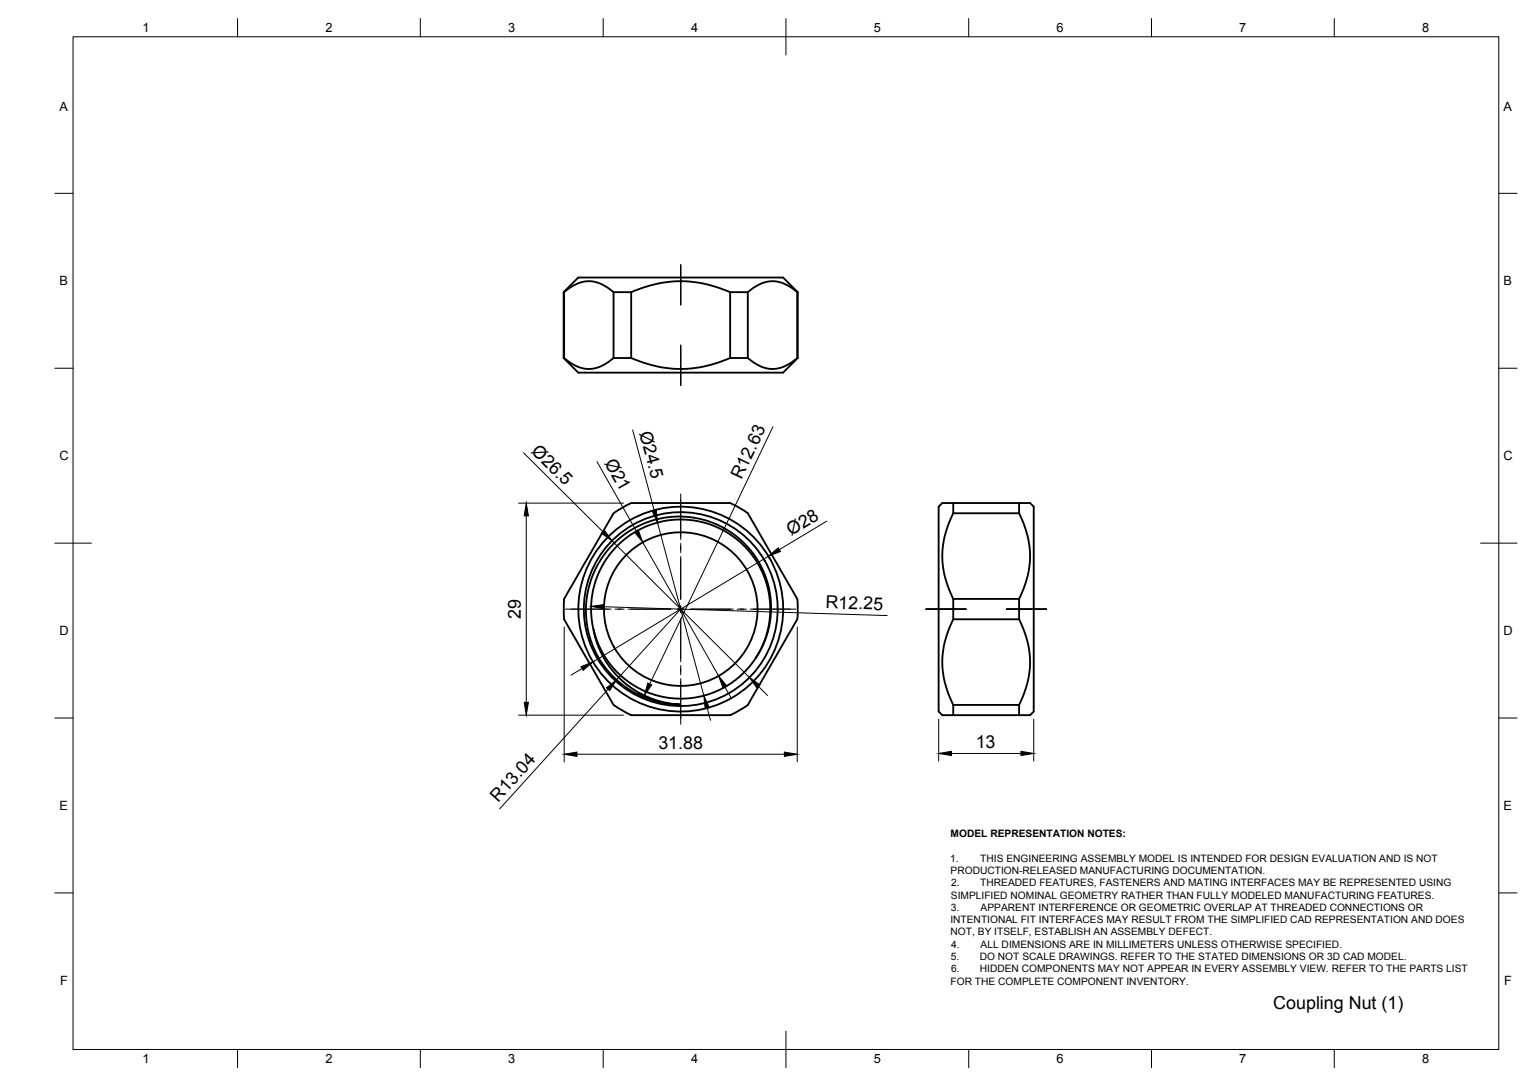
ISO-10303-21;
HEADER;
/* Generated by software containing ST-Developer
 * from STEP Tools, Inc. (www.steptools.com) 
 */

FILE_DESCRIPTION(
/* description */ ('STEP AP214'),
/* implementation_level */ '2;1');

FILE_NAME(
/* name */ 'Coupling Nut (1).step',
/* time_stamp */ '2026-10-05T23:18:41-07:00',
/* author */ (''),
/* organization */ (''),
/* preprocessor_version */ 'ST-DEVELOPER v20.2',
/* originating_system */ 'Autodesk Translation Framework v15.15.0.0',
/* authorisation */ '');

FILE_SCHEMA (('AUTOMOTIVE_DESIGN { 1 0 10303 214 3 1 1 }'));
ENDSEC;

DATA;
#10=MECHANICAL_DESIGN_GEOMETRIC_PRESENTATION_REPRESENTATION('',(#107),#221662);
#69=MANIFOLD_SOLID_BREP('Body1',#79329);
#81=SHAPE_REPRESENTATION_RELATIONSHIP('SRR','None',#221716,#94);
#94=ADVANCED_BREP_SHAPE_REPRESENTATION('',(#69),#221656);
#107=STYLED_ITEM('',(#221783),#69);
#191=B_SPLINE_SURFACE_WITH_KNOTS('',3,3,((#179610,#179611,#179612,#179613,
#179614,#179615,#179616,#179617,#179618,#179619,#179620,#179621,#179622,
#179623,#179624,#179625,#179626,#179627,#179628,#179629,#179630,#179631,
#179632,#179633,#179634,#179635,#179636,#179637,#179638,#179639,#179640,
#179641,#179642,#179643,#179644),(#179645,#179646,#179647,#179648,#179649,
#179650,#179651,#179652,#179653,#179654,#179655,#179656,#179657,#179658,
#179659,#179660,#179661,#179662,#179663,#179664,#179665,#179666,#179667,
#179668,#179669,#179670,#179671,#179672,#179673,#179674,#179675,#179676,
#179677,#179678,#179679),(#179680,#179681,#179682,#179683,#179684,#179685,
#179686,#179687,#179688,#179689,#179690,#179691,#179692,#179693,#179694,
#179695,#179696,#179697,#179698,#179699,#179700,#179701,#179702,#179703,
#179704,#179705,#179706,#179707,#179708,#179709,#179710,#179711,#179712,
#179713,#179714),(#179715,#179716,#179717,#179718,#179719,#179720,#179721,
#179722,#179723,#179724,#179725,#179726,#179727,#179728,#179729,#179730,
#179731,#179732,#179733,#179734,#179735,#179736,#179737,#179738,#179739,
#179740,#179741,#179742,#179743,#179744,#179745,#179746,#179747,#179748,
#179749)),.UNSPECIFIED.,.F.,.F.,.F.,(4,4),(4,1,1,1,1,1,1,1,1,1,1,1,1,1,
1,1,1,1,1,1,1,1,1,1,1,1,1,1,1,1,1,1,4),(0.,1.),(0.,0.031249999999992,0.062499999999984,
0.0937500000001036,0.125000000000096,0.156250000000088,0.187500000000079,
0.218750000000072,0.250000000000191,0.281250000000183,0.312500000000176,
0.343750000000167,0.375000000000159,0.406250000000151,0.437500000000271,
0.468750000000263,0.500000000000255,0.531250000000247,0.562500000000239,
0.593750000000231,0.62500000000035,0.656250000000342,0.687500000000335,
0.718750000000326,0.750000000000319,0.781250000000438,0.81250000000043,
0.843750000000422,0.875000000000414,0.906250000000406,0.937500000000398,
0.968750000000518,1.),.UNSPECIFIED.);
#192=B_SPLINE_SURFACE_WITH_KNOTS('',3,3,((#180017,#180018,#180019,#180020,
#180021,#180022,#180023,#180024,#180025,#180026,#180027,#180028,#180029,
#180030,#180031,#180032,#180033,#180034,#180035,#180036,#180037,#180038,
#180039,#180040,#180041,#180042,#180043,#180044,#180045,#180046,#180047,
#180048,#180049,#180050,#180051),(#180052,#180053,#180054,#180055,#180056,
#180057,#180058,#180059,#180060,#180061,#180062,#180063,#180064,#180065,
#180066,#180067,#180068,#180069,#180070,#180071,#180072,#180073,#180074,
#180075,#180076,#180077,#180078,#180079,#180080,#180081,#180082,#180083,
#180084,#180085,#180086),(#180087,#180088,#180089,#180090,#180091,#180092,
#180093,#180094,#180095,#180096,#180097,#180098,#180099,#180100,#180101,
#180102,#180103,#180104,#180105,#180106,#180107,#180108,#180109,#180110,
#180111,#180112,#180113,#180114,#180115,#180116,#180117,#180118,#180119,
#180120,#180121),(#180122,#180123,#180124,#180125,#180126,#180127,#180128,
#180129,#180130,#180131,#180132,#180133,#180134,#180135,#180136,#180137,
#180138,#180139,#180140,#180141,#180142,#180143,#180144,#180145,#180146,
#180147,#180148,#180149,#180150,#180151,#180152,#180153,#180154,#180155,
#180156)),.UNSPECIFIED.,.F.,.F.,.F.,(4,4),(4,1,1,1,1,1,1,1,1,1,1,1,1,1,
1,1,1,1,1,1,1,1,1,1,1,1,1,1,1,1,1,1,4),(0.,1.),(0.,0.031250000000078,0.0625000000000372,
0.0937500000001152,0.125000000000074,0.156250000000034,0.187500000000111,
0.218750000000071,0.250000000000148,0.281250000000108,0.312500000000186,
0.343750000000145,0.375000000000104,0.406250000000182,0.437500000000141,
0.468750000000219,0.500000000000178,0.531250000000256,0.562500000000216,
0.593750000000175,0.625000000000253,0.656250000000212,0.68750000000029,
0.718750000000249,0.750000000000208,0.781250000000286,0.812500000000245,
0.843750000000323,0.875000000000282,0.90625000000036,0.93750000000032,0.968750000000279,
1.),.UNSPECIFIED.);
#193=B_SPLINE_SURFACE_WITH_KNOTS('',3,3,((#180239,#180240,#180241,#180242,
#180243,#180244,#180245,#180246,#180247,#180248,#180249,#180250,#180251,
#180252,#180253,#180254,#180255,#180256,#180257,#180258,#180259,#180260,
#180261,#180262,#180263,#180264,#180265,#180266,#180267,#180268,#180269,
#180270,#180271,#180272,#180273,#180274,#180275,#180276,#180277,#180278,
#180279,#180280,#180281,#180282,#180283,#180284,#180285,#180286,#180287,
#180288,#180289,#180290,#180291,#180292,#180293,#180294,#180295,#180296,
#180297,#180298,#180299,#180300,#180301,#180302,#180303,#180304,#180305),
(#180306,#180307,#180308,#180309,#180310,#180311,#180312,#180313,#180314,
#180315,#180316,#180317,#180318,#180319,#180320,#180321,#180322,#180323,
#180324,#180325,#180326,#180327,#180328,#180329,#180330,#180331,#180332,
#180333,#180334,#180335,#180336,#180337,#180338,#180339,#180340,#180341,
#180342,#180343,#180344,#180345,#180346,#180347,#180348,#180349,#180350,
#180351,#180352,#180353,#180354,#180355,#180356,#180357,#180358,#180359,
#180360,#180361,#180362,#180363,#180364,#180365,#180366,#180367,#180368,
#180369,#180370,#180371,#180372),(#180373,#180374,#180375,#180376,#180377,
#180378,#180379,#180380,#180381,#180382,#180383,#180384,#180385,#180386,
#180387,#180388,#180389,#180390,#180391,#180392,#180393,#180394,#180395,
#180396,#180397,#180398,#180399,#180400,#180401,#180402,#180403,#180404,
#180405,#180406,#180407,#180408,#180409,#180410,#180411,#180412,#180413,
#180414,#180415,#180416,#180417,#180418,#180419,#180420,#180421,#180422,
#180423,#180424,#180425,#180426,#180427,#180428,#180429,#180430,#180431,
#180432,#180433,#180434,#180435,#180436,#180437,#180438,#180439),(#180440,
#180441,#180442,#180443,#180444,#180445,#180446,#180447,#180448,#180449,
#180450,#180451,#180452,#180453,#180454,#180455,#180456,#180457,#180458,
#180459,#180460,#180461,#180462,#180463,#180464,#180465,#180466,#180467,
#180468,#180469,#180470,#180471,#180472,#180473,#180474,#180475,#180476,
#180477,#180478,#180479,#180480,#180481,#180482,#180483,#180484,#180485,
#180486,#180487,#180488,#180489,#180490,#180491,#180492,#180493,#180494,
#180495,#180496,#180497,#180498,#180499,#180500,#180501,#180502,#180503,
#180504,#180505,#180506)),.UNSPECIFIED.,.F.,.F.,.F.,(4,4),(4,1,1,1,1,1,
1,1,1,1,1,1,1,1,1,1,1,1,1,1,1,1,1,1,1,1,1,1,1,1,1,1,1,1,1,1,1,1,1,1,1,1,
1,1,1,1,1,1,1,1,1,1,1,1,1,1,1,1,1,1,1,1,1,1,4),(0.,1.),(0.,0.015625,0.03125,
0.046875,0.0625,0.078125,0.09375,0.109375,0.125,0.140625,0.15625,0.171875,
0.1875,0.203125,0.21875,0.234375,0.25,0.265625,0.28125,0.296875,0.3125,
0.328125,0.34375,0.359375,0.375,0.390625,0.40625,0.421875,0.4375,0.453125,
0.46875,0.484375,0.5,0.515625,0.53125,0.546875,0.5625,0.578125,0.59375,
0.609375,0.625,0.640625,0.65625,0.671875,0.6875,0.703125,0.71875,0.734375,
0.75,0.765625,0.78125,0.796875,0.8125,0.828125,0.84375,0.859375,0.875,0.890625,
0.90625,0.921875,0.9375,0.953125,0.96875,0.984375,1.),.UNSPECIFIED.);
#194=B_SPLINE_SURFACE_WITH_KNOTS('',3,3,((#180514,#180515,#180516,#180517,
#180518),(#180519,#180520,#180521,#180522,#180523),(#180524,#180525,#180526,
#180527,#180528),(#180529,#180530,#180531,#180532,#180533)),
 .UNSPECIFIED.,.F.,.F.,.F.,(4,4),(4,1,4),(0.,1.),(0.,0.500000000000012,
1.),.UNSPECIFIED.);
#195=B_SPLINE_SURFACE_WITH_KNOTS('',3,1,((#180592,#180593),(#180594,#180595),
(#180596,#180597),(#180598,#180599),(#180600,#180601),(#180602,#180603),
(#180604,#180605),(#180606,#180607),(#180608,#180609),(#180610,#180611),
(#180612,#180613),(#180614,#180615)),.UNSPECIFIED.,.F.,.F.,.F.,(4,2,2,2,
2,4),(2,2),(0.0140497253938089,0.25,0.5,0.75,0.875,0.987103459251385),(0.,
0.0717898562567659),.UNSPECIFIED.);
#196=B_SPLINE_SURFACE_WITH_KNOTS('',3,3,((#180674,#180675,#180676,#180677,
#180678),(#180679,#180680,#180681,#180682,#180683),(#180684,#180685,#180686,
#180687,#180688),(#180689,#180690,#180691,#180692,#180693)),
 .UNSPECIFIED.,.F.,.F.,.F.,(4,4),(4,1,4),(0.,1.),(0.,0.500000000000012,
1.),.UNSPECIFIED.);
#197=B_SPLINE_SURFACE_WITH_KNOTS('',3,3,((#180700,#180701,#180702,#180703,
#180704,#180705,#180706,#180707,#180708,#180709,#180710,#180711,#180712,
#180713,#180714,#180715,#180716,#180717,#180718,#180719,#180720,#180721,
#180722,#180723,#180724,#180725,#180726,#180727,#180728,#180729,#180730,
#180731,#180732,#180733,#180734,#180735,#180736,#180737,#180738,#180739,
#180740,#180741,#180742,#180743,#180744,#180745,#180746,#180747,#180748,
#180749,#180750,#180751,#180752,#180753,#180754,#180755,#180756,#180757,
#180758,#180759,#180760,#180761,#180762,#180763,#180764,#180765,#180766),
(#180767,#180768,#180769,#180770,#180771,#180772,#180773,#180774,#180775,
#180776,#180777,#180778,#180779,#180780,#180781,#180782,#180783,#180784,
#180785,#180786,#180787,#180788,#180789,#180790,#180791,#180792,#180793,
#180794,#180795,#180796,#180797,#180798,#180799,#180800,#180801,#180802,
#180803,#180804,#180805,#180806,#180807,#180808,#180809,#180810,#180811,
#180812,#180813,#180814,#180815,#180816,#180817,#180818,#180819,#180820,
#180821,#180822,#180823,#180824,#180825,#180826,#180827,#180828,#180829,
#180830,#180831,#180832,#180833),(#180834,#180835,#180836,#180837,#180838,
#180839,#180840,#180841,#180842,#180843,#180844,#180845,#180846,#180847,
#180848,#180849,#180850,#180851,#180852,#180853,#180854,#180855,#180856,
#180857,#180858,#180859,#180860,#180861,#180862,#180863,#180864,#180865,
#180866,#180867,#180868,#180869,#180870,#180871,#180872,#180873,#180874,
#180875,#180876,#180877,#180878,#180879,#180880,#180881,#180882,#180883,
#180884,#180885,#180886,#180887,#180888,#180889,#180890,#180891,#180892,
#180893,#180894,#180895,#180896,#180897,#180898,#180899,#180900),(#180901,
#180902,#180903,#180904,#180905,#180906,#180907,#180908,#180909,#180910,
#180911,#180912,#180913,#180914,#180915,#180916,#180917,#180918,#180919,
#180920,#180921,#180922,#180923,#180924,#180925,#180926,#180927,#180928,
#180929,#180930,#180931,#180932,#180933,#180934,#180935,#180936,#180937,
#180938,#180939,#180940,#180941,#180942,#180943,#180944,#180945,#180946,
#180947,#180948,#180949,#180950,#180951,#180952,#180953,#180954,#180955,
#180956,#180957,#180958,#180959,#180960,#180961,#180962,#180963,#180964,
#180965,#180966,#180967)),.UNSPECIFIED.,.F.,.F.,.F.,(4,4),(4,1,1,1,1,1,
1,1,1,1,1,1,1,1,1,1,1,1,1,1,1,1,1,1,1,1,1,1,1,1,1,1,1,1,1,1,1,1,1,1,1,1,
1,1,1,1,1,1,1,1,1,1,1,1,1,1,1,1,1,1,1,1,1,1,4),(0.,1.),(0.,0.015625,0.03125,
0.046875,0.0625,0.078125,0.09375,0.109375,0.125,0.140625,0.15625,0.171875,
0.1875,0.203125,0.21875,0.234375,0.25,0.265625,0.28125,0.296875,0.3125,
0.328125,0.34375,0.359375,0.375,0.390625,0.40625,0.421875,0.4375,0.453125,
0.46875,0.484375,0.5,0.515625,0.53125,0.546875,0.5625,0.578125,0.59375,
0.609375,0.625,0.640625,0.65625,0.671875,0.6875,0.703125,0.71875,0.734375,
0.75,0.765625,0.78125,0.796875,0.8125,0.828125,0.84375,0.859375,0.875,0.890625,
0.90625,0.921875,0.9375,0.953125,0.96875,0.984375,1.),.UNSPECIFIED.);
#198=B_SPLINE_SURFACE_WITH_KNOTS('',3,3,((#180968,#180969,#180970,#180971,
#180972,#180973,#180974,#180975,#180976,#180977,#180978,#180979,#180980,
#180981,#180982,#180983,#180984,#180985,#180986,#180987,#180988,#180989,
#180990,#180991,#180992,#180993,#180994,#180995,#180996,#180997,#180998,
#180999,#181000,#181001,#181002),(#181003,#181004,#181005,#181006,#181007,
#181008,#181009,#181010,#181011,#181012,#181013,#181014,#181015,#181016,
#181017,#181018,#181019,#181020,#181021,#181022,#181023,#181024,#181025,
#181026,#181027,#181028,#181029,#181030,#181031,#181032,#181033,#181034,
#181035,#181036,#181037),(#181038,#181039,#181040,#181041,#181042,#181043,
#181044,#181045,#181046,#181047,#181048,#181049,#181050,#181051,#181052,
#181053,#181054,#181055,#181056,#181057,#181058,#181059,#181060,#181061,
#181062,#181063,#181064,#181065,#181066,#181067,#181068,#181069,#181070,
#181071,#181072),(#181073,#181074,#181075,#181076,#181077,#181078,#181079,
#181080,#181081,#181082,#181083,#181084,#181085,#181086,#181087,#181088,
#181089,#181090,#181091,#181092,#181093,#181094,#181095,#181096,#181097,
#181098,#181099,#181100,#181101,#181102,#181103,#181104,#181105,#181106,
#181107)),.UNSPECIFIED.,.F.,.F.,.F.,(4,4),(4,1,1,1,1,1,1,1,1,1,1,1,1,1,
1,1,1,1,1,1,1,1,1,1,1,1,1,1,1,1,1,1,4),(0.,1.),(0.,0.031250000000078,0.0625000000000372,
0.0937500000001152,0.125000000000074,0.156250000000034,0.187500000000111,
0.218750000000071,0.250000000000148,0.281250000000108,0.312500000000186,
0.343750000000145,0.375000000000104,0.406250000000182,0.437500000000141,
0.468750000000219,0.500000000000178,0.531250000000256,0.562500000000216,
0.593750000000175,0.625000000000253,0.656250000000212,0.68750000000029,
0.718750000000249,0.750000000000208,0.781250000000286,0.812500000000245,
0.843750000000323,0.875000000000282,0.90625000000036,0.93750000000032,0.968750000000279,
1.),.UNSPECIFIED.);
#302=FACE_BOUND('',#24853,.T.);
#303=FACE_BOUND('',#24863,.T.);
#304=FACE_BOUND('',#24865,.T.);
#1788=(
BOUNDED_CURVE()
B_SPLINE_CURVE(2,(#179504,#179505,#179506),.UNSPECIFIED.,.F.,.F.)
B_SPLINE_CURVE_WITH_KNOTS((3,3),(1.60808462077176,3.73981215786377),
 .UNSPECIFIED.)
CURVE()
GEOMETRIC_REPRESENTATION_ITEM()
RATIONAL_B_SPLINE_CURVE((1.37704917963476,1.51950254302061,1.37704917962903))
REPRESENTATION_ITEM('')
);
#1789=(
BOUNDED_CURVE()
B_SPLINE_CURVE(2,(#179510,#179511,#179512),.UNSPECIFIED.,.F.,.F.)
B_SPLINE_CURVE_WITH_KNOTS((3,3),(1.608096434994,3.73983031850901),
 .UNSPECIFIED.)
CURVE()
GEOMETRIC_REPRESENTATION_ITEM()
RATIONAL_B_SPLINE_CURVE((1.37705242397046,1.51950612297584,1.37705242396616))
REPRESENTATION_ITEM('')
);
#1790=(
BOUNDED_CURVE()
B_SPLINE_CURVE(2,(#179516,#179517,#179518),.UNSPECIFIED.,.F.,.F.)
B_SPLINE_CURVE_WITH_KNOTS((3,3),(-3.73983031850899,-1.60809643499399),
 .UNSPECIFIED.)
CURVE()
GEOMETRIC_REPRESENTATION_ITEM()
RATIONAL_B_SPLINE_CURVE((1.37705242396616,1.51950612297584,1.37705242397046))
REPRESENTATION_ITEM('')
);
#1791=(
BOUNDED_CURVE()
B_SPLINE_CURVE(2,(#179522,#179523,#179524),.UNSPECIFIED.,.F.,.F.)
B_SPLINE_CURVE_WITH_KNOTS((3,3),(1.60808462077176,3.73981215785304),
 .UNSPECIFIED.)
CURVE()
GEOMETRIC_REPRESENTATION_ITEM()
RATIONAL_B_SPLINE_CURVE((1.37704917963476,1.51950254301988,1.37704917963046))
REPRESENTATION_ITEM('')
);
#1792=(
BOUNDED_CURVE()
B_SPLINE_CURVE(2,(#179528,#179529,#179530),.UNSPECIFIED.,.F.,.F.)
B_SPLINE_CURVE_WITH_KNOTS((3,3),(1.60809643499362,3.73983031850844),
 .UNSPECIFIED.)
CURVE()
GEOMETRIC_REPRESENTATION_ITEM()
RATIONAL_B_SPLINE_CURVE((1.37705242397036,1.51950612297573,1.37705242396606))
REPRESENTATION_ITEM('')
);
#1793=(
BOUNDED_CURVE()
B_SPLINE_CURVE(2,(#179539,#179540,#179541),.UNSPECIFIED.,.F.,.F.)
B_SPLINE_CURVE_WITH_KNOTS((3,3),(1.60809643499432,3.73983031850951),
 .UNSPECIFIED.)
CURVE()
GEOMETRIC_REPRESENTATION_ITEM()
RATIONAL_B_SPLINE_CURVE((1.37705242397056,1.51950612297595,1.37705242396626))
REPRESENTATION_ITEM('')
);
#1794=(
BOUNDED_CURVE()
B_SPLINE_CURVE(2,(#179546,#179547,#179548),.UNSPECIFIED.,.F.,.F.)
B_SPLINE_CURVE_WITH_KNOTS((3,3),(1.76947846838519,3.98831685496984),
 .UNSPECIFIED.)
CURVE()
GEOMETRIC_REPRESENTATION_ITEM()
RATIONAL_B_SPLINE_CURVE((1.4216188517591,1.56868287088004,1.4216188517602))
REPRESENTATION_ITEM('')
);
#1795=(
BOUNDED_CURVE()
B_SPLINE_CURVE(2,(#179552,#179553,#179554),.UNSPECIFIED.,.F.,.F.)
B_SPLINE_CURVE_WITH_KNOTS((3,3),(-3.98831685495251,-1.76947846838546),
 .UNSPECIFIED.)
CURVE()
GEOMETRIC_REPRESENTATION_ITEM()
RATIONAL_B_SPLINE_CURVE((1.42161885176135,1.56868287087821,1.42161885175877))
REPRESENTATION_ITEM('')
);
#1796=(
BOUNDED_CURVE()
B_SPLINE_CURVE(2,(#179558,#179559,#179560),.UNSPECIFIED.,.F.,.F.)
B_SPLINE_CURVE_WITH_KNOTS((3,3),(1.76947846838545,3.98831685495252),
 .UNSPECIFIED.)
CURVE()
GEOMETRIC_REPRESENTATION_ITEM()
RATIONAL_B_SPLINE_CURVE((1.42161885175877,1.56868287087821,1.42161885176135))
REPRESENTATION_ITEM('')
);
#1797=(
BOUNDED_CURVE()
B_SPLINE_CURVE(2,(#179564,#179565,#179566),.UNSPECIFIED.,.F.,.F.)
B_SPLINE_CURVE_WITH_KNOTS((3,3),(1.76947846838366,3.98831685496743),
 .UNSPECIFIED.)
CURVE()
GEOMETRIC_REPRESENTATION_ITEM()
RATIONAL_B_SPLINE_CURVE((1.42161885175867,1.56868287087956,1.42161885175977))
REPRESENTATION_ITEM('')
);
#1798=(
BOUNDED_CURVE()
B_SPLINE_CURVE(2,(#179570,#179571,#179572),.UNSPECIFIED.,.F.,.F.)
B_SPLINE_CURVE_WITH_KNOTS((3,3),(-3.98831685495253,-1.76947846838542),
 .UNSPECIFIED.)
CURVE()
GEOMETRIC_REPRESENTATION_ITEM()
RATIONAL_B_SPLINE_CURVE((1.42161885176134,1.56868287087821,1.42161885175876))
REPRESENTATION_ITEM('')
);
#1799=(
BOUNDED_CURVE()
B_SPLINE_CURVE(2,(#179581,#179582,#179583),.UNSPECIFIED.,.F.,.F.)
B_SPLINE_CURVE_WITH_KNOTS((3,3),(-3.98831685495253,-1.76947846838542),
 .UNSPECIFIED.)
CURVE()
GEOMETRIC_REPRESENTATION_ITEM()
RATIONAL_B_SPLINE_CURVE((1.42161885176135,1.56868287087821,1.42161885175877))
REPRESENTATION_ITEM('')
);
#1944=CONICAL_SURFACE('',#80813,12.750003108,0.785398266415682);
#1945=CONICAL_SURFACE('',#80815,15.,0.7853981625);
#1946=CONICAL_SURFACE('',#80824,15.,0.7853981625);
#2237=CYLINDRICAL_SURFACE('',#80797,13.0486498132185);
#2238=CYLINDRICAL_SURFACE('',#80798,13.0486498132185);
#2239=CYLINDRICAL_SURFACE('',#80799,13.0486498132185);
#2240=CYLINDRICAL_SURFACE('',#80800,12.25);
#2241=CYLINDRICAL_SURFACE('',#80802,12.25);
#2242=CYLINDRICAL_SURFACE('',#80803,12.25);
#2243=CYLINDRICAL_SURFACE('',#80804,12.25);
#2244=CYLINDRICAL_SURFACE('',#80805,12.25);
#2245=CYLINDRICAL_SURFACE('',#80807,10.5);
#2246=CYLINDRICAL_SURFACE('',#80810,12.25);
#2247=CYLINDRICAL_SURFACE('',#80812,13.0486498132185);
#2248=CYLINDRICAL_SURFACE('',#80833,16.);
#2249=CYLINDRICAL_SURFACE('',#80837,16.);
#2250=CYLINDRICAL_SURFACE('',#80838,16.);
#2251=CYLINDRICAL_SURFACE('',#80841,16.);
#2252=CYLINDRICAL_SURFACE('',#80842,16.);
#2253=CYLINDRICAL_SURFACE('',#80843,16.);
#3159=LINE('',#177999,#10226);
#3160=LINE('',#178079,#10227);
#3161=LINE('',#178155,#10228);
#3162=LINE('',#178321,#10229);
#3163=LINE('',#178351,#10230);
#3164=LINE('',#178420,#10231);
#3165=LINE('',#178487,#10232);
#3166=LINE('',#178570,#10233);
#3167=LINE('',#178736,#10234);
#3168=LINE('',#178905,#10235);
#3169=LINE('',#179064,#10236);
#3170=LINE('',#179079,#10237);
#3171=LINE('',#179394,#10238);
#3172=LINE('',#179534,#10239);
#3173=LINE('',#179576,#10240);
#3174=LINE('',#179586,#10241);
#3175=LINE('',#179587,#10242);
#3176=LINE('',#179589,#10243);
#3177=LINE('',#179590,#10244);
#3178=LINE('',#179592,#10245);
#3179=LINE('',#179594,#10246);
#3180=LINE('',#179596,#10247);
#3181=LINE('',#179598,#10248);
#3182=LINE('',#179600,#10249);
#3183=LINE('',#179602,#10250);
#3184=LINE('',#179603,#10251);
#3185=LINE('',#179606,#10252);
#3186=LINE('',#180016,#10253);
#3187=LINE('',#180513,#10254);
#10226=VECTOR('',#89254,13.0486498132185);
#10227=VECTOR('',#89255,10.);
#10228=VECTOR('',#89258,13.0486498132185);
#10229=VECTOR('',#89261,13.0486498132185);
#10230=VECTOR('',#89264,12.25);
#10231=VECTOR('',#89265,10.);
#10232=VECTOR('',#89266,12.25);
#10233=VECTOR('',#89271,12.25);
#10234=VECTOR('',#89274,12.25);
#10235=VECTOR('',#89277,12.25);
#10236=VECTOR('',#89280,12.25);
#10237=VECTOR('',#89287,10.5);
#10238=VECTOR('',#89298,12.750003108);
#10239=VECTOR('',#89313,15.);
#10240=VECTOR('',#89332,15.);
#10241=VECTOR('',#89341,1000.);
#10242=VECTOR('',#89342,1000.);
#10243=VECTOR('',#89345,1000.);
#10244=VECTOR('',#89346,1000.);
#10245=VECTOR('',#89349,1000.);
#10246=VECTOR('',#89352,1000.);
#10247=VECTOR('',#89355,1000.);
#10248=VECTOR('',#89358,1000.);
#10249=VECTOR('',#89361,1000.);
#10250=VECTOR('',#89364,1000.);
#10251=VECTOR('',#89365,1000.);
#10252=VECTOR('',#89370,1000.);
#10253=VECTOR('',#89377,10.);
#10254=VECTOR('',#89378,10.);
#16994=PLANE('',#80834);
#16995=PLANE('',#80835);
#16996=PLANE('',#80836);
#16997=PLANE('',#80839);
#16998=PLANE('',#80840);
#16999=PLANE('',#80844);
#17000=PLANE('',#80845);
#17001=PLANE('',#80846);
#17002=PLANE('',#80847);
#20754=FACE_OUTER_BOUND('',#24826,.T.);
#20755=FACE_OUTER_BOUND('',#24827,.T.);
#20756=FACE_OUTER_BOUND('',#24828,.T.);
#20757=FACE_OUTER_BOUND('',#24829,.T.);
#20758=FACE_OUTER_BOUND('',#24830,.T.);
#20759=FACE_OUTER_BOUND('',#24831,.T.);
#20760=FACE_OUTER_BOUND('',#24832,.T.);
#20761=FACE_OUTER_BOUND('',#24833,.T.);
#20762=FACE_OUTER_BOUND('',#24834,.T.);
#20763=FACE_OUTER_BOUND('',#24835,.T.);
#20764=FACE_OUTER_BOUND('',#24836,.T.);
#20765=FACE_OUTER_BOUND('',#24837,.T.);
#20766=FACE_OUTER_BOUND('',#24838,.T.);
#20767=FACE_OUTER_BOUND('',#24839,.T.);
#20768=FACE_OUTER_BOUND('',#24840,.T.);
#20769=FACE_OUTER_BOUND('',#24841,.T.);
#20770=FACE_OUTER_BOUND('',#24842,.T.);
#20771=FACE_OUTER_BOUND('',#24843,.T.);
#20772=FACE_OUTER_BOUND('',#24844,.T.);
#20773=FACE_OUTER_BOUND('',#24845,.T.);
#20774=FACE_OUTER_BOUND('',#24846,.T.);
#20775=FACE_OUTER_BOUND('',#24847,.T.);
#20776=FACE_OUTER_BOUND('',#24848,.T.);
#20777=FACE_OUTER_BOUND('',#24849,.T.);
#20778=FACE_OUTER_BOUND('',#24850,.T.);
#20779=FACE_OUTER_BOUND('',#24851,.T.);
#20780=FACE_OUTER_BOUND('',#24852,.T.);
#20781=FACE_OUTER_BOUND('',#24854,.T.);
#20782=FACE_OUTER_BOUND('',#24855,.T.);
#20783=FACE_OUTER_BOUND('',#24856,.T.);
#20784=FACE_OUTER_BOUND('',#24857,.T.);
#20785=FACE_OUTER_BOUND('',#24858,.T.);
#20786=FACE_OUTER_BOUND('',#24859,.T.);
#20787=FACE_OUTER_BOUND('',#24860,.T.);
#20788=FACE_OUTER_BOUND('',#24861,.T.);
#20789=FACE_OUTER_BOUND('',#24862,.T.);
#20790=FACE_OUTER_BOUND('',#24864,.T.);
#24826=EDGE_LOOP('',(#56697,#56698,#56699,#56700,#56701));
#24827=EDGE_LOOP('',(#56702,#56703,#56704,#56705));
#24828=EDGE_LOOP('',(#56706,#56707,#56708,#56709));
#24829=EDGE_LOOP('',(#56710,#56711,#56712,#56713,#56714,#56715,#56716,#56717,
#56718,#56719,#56720,#56721));
#24830=EDGE_LOOP('',(#56722,#56723,#56724,#56725));
#24831=EDGE_LOOP('',(#56726,#56727,#56728,#56729,#56730));
#24832=EDGE_LOOP('',(#56731,#56732,#56733,#56734,#56735));
#24833=EDGE_LOOP('',(#56736,#56737,#56738));
#24834=EDGE_LOOP('',(#56739,#56740,#56741,#56742));
#24835=EDGE_LOOP('',(#56743,#56744,#56745,#56746,#56747,#56748));
#24836=EDGE_LOOP('',(#56749,#56750,#56751,#56752));
#24837=EDGE_LOOP('',(#56753,#56754,#56755,#56756,#56757,#56758,#56759,#56760,
#56761,#56762));
#24838=EDGE_LOOP('',(#56763,#56764,#56765,#56766,#56767,#56768,#56769,#56770,
#56771,#56772,#56773,#56774,#56775,#56776,#56777,#56778));
#24839=EDGE_LOOP('',(#56779,#56780,#56781,#56782,#56783,#56784,#56785,#56786,
#56787,#56788,#56789,#56790,#56791,#56792,#56793,#56794));
#24840=EDGE_LOOP('',(#56795,#56796,#56797,#56798,#56799));
#24841=EDGE_LOOP('',(#56800,#56801,#56802,#56803));
#24842=EDGE_LOOP('',(#56804,#56805,#56806,#56807));
#24843=EDGE_LOOP('',(#56808,#56809,#56810,#56811));
#24844=EDGE_LOOP('',(#56812,#56813,#56814,#56815));
#24845=EDGE_LOOP('',(#56816,#56817,#56818,#56819));
#24846=EDGE_LOOP('',(#56820,#56821,#56822,#56823));
#24847=EDGE_LOOP('',(#56824,#56825,#56826,#56827));
#24848=EDGE_LOOP('',(#56828,#56829,#56830,#56831));
#24849=EDGE_LOOP('',(#56832,#56833,#56834,#56835));
#24850=EDGE_LOOP('',(#56836,#56837,#56838,#56839,#56840));
#24851=EDGE_LOOP('',(#56841,#56842,#56843,#56844));
#24852=EDGE_LOOP('',(#56845));
#24853=EDGE_LOOP('',(#56846));
#24854=EDGE_LOOP('',(#56847,#56848,#56849,#56850,#56851,#56852,#56853));
#24855=EDGE_LOOP('',(#56854,#56855,#56856,#56857,#56858));
#24856=EDGE_LOOP('',(#56859,#56860,#56861,#56862,#56863,#56864,#56865,#56866,
#56867,#56868,#56869));
#24857=EDGE_LOOP('',(#56870,#56871,#56872));
#24858=EDGE_LOOP('',(#56873,#56874,#56875,#56876));
#24859=EDGE_LOOP('',(#56877,#56878,#56879));
#24860=EDGE_LOOP('',(#56880,#56881,#56882,#56883,#56884,#56885,#56886,#56887,
#56888,#56889,#56890,#56891));
#24861=EDGE_LOOP('',(#56892,#56893,#56894,#56895,#56896,#56897,#56898));
#24862=EDGE_LOOP('',(#56899));
#24863=EDGE_LOOP('',(#56900));
#24864=EDGE_LOOP('',(#56901));
#24865=EDGE_LOOP('',(#56902));
#30234=B_SPLINE_CURVE_WITH_KNOTS('',3,(#178001,#178002,#178003,#178004,
#178005,#178006,#178007,#178008,#178009,#178010,#178011,#178012,#178013,
#178014,#178015,#178016,#178017,#178018,#178019,#178020,#178021,#178022,
#178023,#178024,#178025,#178026,#178027,#178028,#178029,#178030,#178031,
#178032,#178033,#178034,#178035,#178036,#178037,#178038,#178039,#178040,
#178041,#178042),.UNSPECIFIED.,.F.,.F.,(4,2,2,2,2,2,2,2,2,2,2,2,2,2,2,2,
2,2,2,2,4),(16.411939559148,16.5276993648978,16.7898103993412,16.9146234716417,
17.1336164713817,17.331869283095,17.5558277390514,17.7571272017244,17.9098817122033,
18.1686635086661,18.3330413380558,18.5331993144161,18.7925278924566,19.0512622565918,
19.1783118587244,19.3819635677508,19.6487024603407,19.7552464035092,20.0145823158284,
20.2601584579687,20.5148551545717),.UNSPECIFIED.);
#30235=B_SPLINE_CURVE_WITH_KNOTS('',3,(#178044,#178045,#178046,#178047,
#178048,#178049,#178050,#178051,#178052,#178053,#178054,#178055,#178056,
#178057,#178058,#178059,#178060,#178061,#178062,#178063,#178064,#178065,
#178066,#178067,#178068,#178069,#178070,#178071,#178072,#178073,#178074,
#178075,#178076,#178077),.UNSPECIFIED.,.F.,.F.,(4,2,2,2,2,2,2,2,2,2,2,2,
2,2,2,2,4),(-3.64743130453341,-3.33257853567476,-3.22780382457832,-2.94609671661996,
-2.68640335637872,-2.43382900975111,-2.07865629233289,-1.823297444294,-1.69779781578983,
-1.49131358643798,-1.2705775614283,-1.11563261310354,-0.884376073702807,
-0.690814598996595,-0.518873862852227,-0.260515535699254,-0.000141823912015393),
 .UNSPECIFIED.);
#30236=B_SPLINE_CURVE_WITH_KNOTS('',3,(#178080,#178081,#178082,#178083,
#178084,#178085,#178086,#178087,#178088,#178089,#178090,#178091,#178092,
#178093,#178094,#178095,#178096,#178097,#178098,#178099,#178100,#178101,
#178102,#178103,#178104,#178105,#178106,#178107,#178108,#178109,#178110,
#178111,#178112,#178113,#178114,#178115,#178116,#178117,#178118,#178119,
#178120,#178121,#178122,#178123,#178124,#178125,#178126,#178127,#178128,
#178129,#178130,#178131,#178132,#178133,#178134,#178135,#178136,#178137,
#178138,#178139,#178140,#178141,#178142,#178143,#178144,#178145,#178146,
#178147,#178148,#178149,#178150,#178151),.UNSPECIFIED.,.F.,.F.,(4,2,2,2,
2,2,2,2,2,2,2,2,2,2,2,2,2,2,2,2,2,2,2,2,2,2,2,2,2,2,2,2,2,2,2,4),(0.000165493788789278,
0.133572515359782,0.265070417066448,0.525261541659564,0.718250836461765,
0.939262619734119,1.10101308860442,1.36078600247732,1.61438552821345,1.86608480335074,
2.10918592858206,2.36534540858103,2.49037418921662,2.71408475481147,2.97308494587933,
3.09890243561411,3.35779973017724,3.57542031480175,3.79208623060398,4.04882373567806,
4.30051979229931,4.55920852636254,4.81123563101406,5.01845678813855,5.27455044290403,
5.52645653972308,5.76250743234395,6.00874266289446,6.20633919438028,6.3337050145735,
6.59244105306261,6.85126540653577,7.05793450067292,7.31164686257427,7.56543499053437,
7.75024417698323),.UNSPECIFIED.);
#30237=B_SPLINE_CURVE_WITH_KNOTS('',3,(#178156,#178157,#178158,#178159,
#178160,#178161,#178162,#178163,#178164,#178165,#178166,#178167,#178168,
#178169,#178170,#178171,#178172,#178173,#178174,#178175,#178176,#178177,
#178178,#178179,#178180,#178181,#178182,#178183,#178184,#178185,#178186,
#178187,#178188,#178189,#178190,#178191,#178192,#178193,#178194,#178195,
#178196,#178197,#178198,#178199,#178200,#178201,#178202,#178203,#178204,
#178205,#178206,#178207,#178208,#178209,#178210,#178211,#178212,#178213,
#178214,#178215,#178216,#178217,#178218,#178219,#178220,#178221,#178222,
#178223,#178224,#178225,#178226,#178227,#178228,#178229,#178230,#178231,
#178232,#178233,#178234,#178235,#178236,#178237),.UNSPECIFIED.,.F.,.F.,
(4,2,2,2,2,2,2,2,2,2,2,2,2,2,2,2,2,2,2,2,2,2,2,2,2,2,2,2,2,2,2,2,2,2,2,
2,2,2,2,2,4),(8.20599054997932,8.35079045388701,8.60924481411329,8.75465398952731,
8.95626211349646,9.21554237835956,9.34443315214084,9.58153550224463,9.77860946937124,
10.0041117166618,10.2579350567844,10.3824872891584,10.6879416879749,10.8130137052272,
11.0351748170972,11.2420075009466,11.4004731687472,11.6129596147629,11.8470240825678,
12.0601025163729,12.2237306704323,12.4823623009414,12.6947479399234,12.8195512556543,
13.0784335443201,13.3076522799465,13.4323904647595,13.6664221203585,13.8636547400886,
14.0842574617044,14.3120516628972,14.5550127212924,14.8073205727347,15.0605117862674,
15.3202978529829,15.4883699770317,15.7022609398385,15.8985108557244,16.1077929373567,
16.3226600726361,16.411939559148),.UNSPECIFIED.);
#30238=B_SPLINE_CURVE_WITH_KNOTS('',3,(#178238,#178239,#178240,#178241,
#178242,#178243,#178244,#178245,#178246,#178247,#178248,#178249,#178250,
#178251,#178252,#178253,#178254,#178255,#178256,#178257,#178258,#178259,
#178260,#178261,#178262,#178263,#178264,#178265,#178266,#178267,#178268,
#178269,#178270,#178271,#178272,#178273,#178274,#178275,#178276,#178277,
#178278,#178279,#178280,#178281,#178282,#178283,#178284,#178285,#178286,
#178287,#178288,#178289,#178290,#178291,#178292,#178293,#178294,#178295,
#178296,#178297,#178298,#178299,#178300,#178301,#178302,#178303,#178304,
#178305,#178306,#178307,#178308,#178309,#178310,#178311,#178312,#178313,
#178314,#178315,#178316,#178317),.UNSPECIFIED.,.F.,.F.,(4,2,2,2,2,2,2,2,
2,2,2,2,2,2,2,2,2,2,2,2,2,2,2,2,2,2,2,2,2,2,2,2,2,2,2,2,2,2,2,4),(7.75024417698323,
7.82451593103171,8.02113898697175,8.28067309482283,8.53374289089235,8.78755898378574,
9.04712635066033,9.26728651955331,9.48617872391405,9.68037806711142,9.90991948493791,
10.0351210994055,10.2947590347315,10.4947121782736,10.7212623316305,10.8466717851503,
11.1058046174447,11.3157786202329,11.5462098319442,11.6980972601113,11.9564972275347,
12.0809855194537,12.3324431280832,12.5428274659398,12.7594848200696,13.0187426511126,
13.2711191413954,13.5240636571919,13.7831182451389,13.9451540287318,14.1483747254047,
14.4416992472351,14.5664190762602,14.7966381602951,14.9957380443166,15.260658195038,
15.3855066671222,15.5901676955325,15.848864838421,15.9563811041735),
 .UNSPECIFIED.);
#30239=B_SPLINE_CURVE_WITH_KNOTS('',3,(#178323,#178324,#178325,#178326,
#178327,#178328,#178329,#178330,#178331,#178332),.UNSPECIFIED.,.F.,.F.,
(4,2,2,2,4),(0.000122513986806074,0.222884378529465,0.446676969347694,0.675563919565001,
0.912296554340542),.UNSPECIFIED.);
#30240=B_SPLINE_CURVE_WITH_KNOTS('',3,(#178334,#178335,#178336,#178337),
 .UNSPECIFIED.,.F.,.F.,(4,4),(0.,1.),.UNSPECIFIED.);
#30241=B_SPLINE_CURVE_WITH_KNOTS('',3,(#178338,#178339,#178340,#178341,
#178342,#178343,#178344,#178345,#178346,#178347),.UNSPECIFIED.,.F.,.F.,
(4,2,2,2,4),(-0.912452539736376,-0.684829823365645,-0.456379958242787,-0.343466785291317,
-6.86284440253819E-5),.UNSPECIFIED.);
#30242=B_SPLINE_CURVE_WITH_KNOTS('',3,(#178353,#178354,#178355,#178356,
#178357,#178358,#178359,#178360,#178361,#178362,#178363,#178364,#178365,
#178366,#178367,#178368,#178369,#178370,#178371,#178372,#178373,#178374,
#178375,#178376,#178377,#178378,#178379,#178380,#178381,#178382,#178383,
#178384,#178385,#178386,#178387,#178388,#178389,#178390,#178391,#178392,
#178393,#178394,#178395,#178396),.UNSPECIFIED.,.F.,.F.,(4,2,2,2,2,2,2,2,
2,2,2,2,2,2,2,2,2,2,2,2,2,4),(-3.85203272472586,-3.81068214158194,-3.60033621336808,
-3.48309143663605,-3.23993317549133,-3.0806350821531,-2.83736961014879,
-2.72030932217897,-2.47717399183909,-2.32489351843059,-2.08166265518047,
-1.96051566916432,-1.71743905866922,-1.44667552022466,-1.3282758343242,
-1.17213639367387,-0.928887044086265,-0.812271660099406,-0.610350351616681,
-0.31037347820266,-0.156424378504126,-9.99999996142975E-7),
 .UNSPECIFIED.);
#30243=B_SPLINE_CURVE_WITH_KNOTS('',3,(#178398,#178399,#178400,#178401,
#178402,#178403,#178404,#178405,#178406,#178407),.UNSPECIFIED.,.F.,.F.,
(4,2,2,2,4),(-0.856199781212238,-0.642101402330389,-0.428204524303658,-0.321759740087186,
0.),.UNSPECIFIED.);
#30244=B_SPLINE_CURVE_WITH_KNOTS('',3,(#178409,#178410,#178411,#178412,
#178413,#178414,#178415,#178416,#178417,#178418),.UNSPECIFIED.,.F.,.F.,
(4,2,2,2,4),(-1.24857216709389,-0.938370073705948,-0.624319392609061,-0.31407240746023,
-1.91505823160449E-6),.UNSPECIFIED.);
#30245=B_SPLINE_CURVE_WITH_KNOTS('',3,(#178422,#178423,#178424,#178425,
#178426,#178427,#178428,#178429,#178430,#178431),.UNSPECIFIED.,.F.,.F.,
(4,2,2,2,4),(-1.24672715675234,-0.933142576513486,-0.623377583747118,-0.309803734768733,
-7.91147252940148E-5),.UNSPECIFIED.);
#30246=B_SPLINE_CURVE_WITH_KNOTS('',3,(#178433,#178434,#178435,#178436,
#178437,#178438,#178439,#178440,#178441,#178442),.UNSPECIFIED.,.F.,.F.,
(4,2,2,2,4),(-0.85620344504763,-0.534443747738016,-0.427999096338903,-0.214103034436443,
-6.19686689110128E-6),.UNSPECIFIED.);
#30247=B_SPLINE_CURVE_WITH_KNOTS('',3,(#178444,#178445,#178446,#178447,
#178448,#178449,#178450,#178451,#178452,#178453,#178454,#178455,#178456,
#178457,#178458,#178459,#178460,#178461,#178462,#178463,#178464,#178465,
#178466,#178467,#178468,#178469,#178470,#178471,#178472,#178473,#178474,
#178475,#178476,#178477,#178478,#178479,#178480,#178481,#178482,#178483,
#178484,#178485),.UNSPECIFIED.,.F.,.F.,(4,2,2,2,2,2,2,2,2,2,2,2,2,2,2,2,
2,2,2,2,4),(-22.6856736757846,-22.4729484327686,-22.2608902357116,-22.1224645885887,
-21.9401656304958,-21.6971390197663,-21.5797484468213,-21.3707797129937,
-21.1275346348255,-20.9740534912599,-20.7309072529524,-20.6138113800813,
-20.3705385067576,-20.2109568292684,-19.9677909680696,-19.8232856164035,
-19.5801706501752,-19.4393531223485,-19.1962535931423,-18.9580519542603,
-18.8335546705084),.UNSPECIFIED.);
#30248=B_SPLINE_CURVE_WITH_KNOTS('',3,(#178489,#178490,#178491,#178492,
#178493,#178494,#178495,#178496,#178497,#178498,#178499,#178500,#178501,
#178502,#178503,#178504,#178505,#178506,#178507,#178508,#178509,#178510,
#178511,#178512,#178513,#178514,#178515,#178516,#178517,#178518,#178519,
#178520,#178521,#178522,#178523,#178524,#178525,#178526,#178527,#178528,
#178529,#178530,#178531,#178532,#178533,#178534,#178535,#178536,#178537,
#178538,#178539,#178540,#178541,#178542,#178543,#178544,#178545,#178546,
#178547,#178548,#178549,#178550,#178551,#178552,#178553,#178554,#178555,
#178556,#178557,#178558,#178559,#178560,#178561,#178562,#178563,#178564,
#178565,#178566),.UNSPECIFIED.,.F.,.F.,(4,2,2,2,2,2,2,2,2,2,2,2,2,2,2,2,
2,2,2,2,2,2,2,2,2,2,2,2,2,2,2,2,2,2,2,2,2,2,4),(-18.8335546705084,-18.7227357997547,
-18.4794804275072,-18.3029946229965,-18.0597884772514,-17.9421642824665,
-17.6988795154385,-17.5345187053728,-17.2913374272366,-17.1457737280561,
-16.9026517389328,-16.6642788314431,-16.3365927448224,-16.2192214989655,
-15.9859590265659,-15.7503815683893,-15.512436383961,-15.2774941236952,
-15.0545123299144,-14.811474357221,-14.6940767755213,-14.4845852214616,
-14.2413335075011,-14.0877730700931,-13.9694005212358,-13.6992966442092,
-13.4562052826424,-13.33505073917,-13.0918047666125,-12.8525232134558,-12.6150000024995,
-12.3718115009665,-12.1843740433989,-11.941143292846,-11.8233203791244,
-11.5800278639557,-11.3420914658496,-11.2248334089522,-11.1284471789905),
 .UNSPECIFIED.);
#30249=B_SPLINE_CURVE_WITH_KNOTS('',3,(#178571,#178572,#178573,#178574,
#178575,#178576,#178577,#178578,#178579,#178580,#178581,#178582,#178583,
#178584,#178585,#178586,#178587,#178588,#178589,#178590,#178591,#178592,
#178593,#178594,#178595,#178596,#178597,#178598,#178599,#178600,#178601,
#178602,#178603,#178604,#178605,#178606,#178607,#178608,#178609,#178610,
#178611,#178612,#178613,#178614,#178615,#178616,#178617,#178618,#178619,
#178620,#178621,#178622,#178623,#178624,#178625,#178626,#178627,#178628,
#178629,#178630,#178631,#178632,#178633,#178634,#178635,#178636,#178637,
#178638,#178639,#178640,#178641,#178642,#178643,#178644,#178645,#178646,
#178647,#178648),.UNSPECIFIED.,.F.,.F.,(4,2,2,2,2,2,2,2,2,2,2,2,2,2,2,2,
2,2,2,2,2,2,2,2,2,2,2,2,2,2,2,2,2,2,2,2,2,2,4),(-11.5566456717678,-11.4598611162991,
-11.3426388598562,-11.1047720742011,-10.8614846878278,-10.7436406873222,
-10.5004129844007,-10.3115727442124,-10.0919136118381,-9.97374824847428,
-9.73049762835425,-9.51862735066146,-9.40121052478211,-9.15814875252158,
-8.93140561123793,-8.6952260136082,-8.45648843501656,-8.21332578494614,
-8.05479937138979,-7.81152977304203,-7.69455898882562,-7.45142845787144,
-7.30240675633191,-7.05919460455083,-6.87747816562279,-6.63427898704334,
-6.39780330111834,-6.15890783331182,-5.91572809274957,-5.74977652524943,
-5.50649627086529,-5.38871321866122,-5.14549760697054,-4.96012413551749,
-4.716995797981,-4.4798366946526,-4.24065538165822,-3.99743850082616,-3.85203272472586),
 .UNSPECIFIED.);
#30250=B_SPLINE_CURVE_WITH_KNOTS('',3,(#178649,#178650,#178651,#178652,
#178653,#178654,#178655,#178656,#178657,#178658,#178659,#178660,#178661,
#178662,#178663,#178664,#178665,#178666,#178667,#178668,#178669,#178670,
#178671,#178672,#178673,#178674,#178675,#178676,#178677,#178678,#178679,
#178680,#178681,#178682,#178683,#178684,#178685,#178686,#178687,#178688,
#178689,#178690,#178691,#178692,#178693,#178694,#178695,#178696,#178697,
#178698,#178699,#178700,#178701,#178702,#178703,#178704,#178705,#178706,
#178707,#178708,#178709,#178710,#178711,#178712,#178713,#178714,#178715,
#178716,#178717,#178718,#178719,#178720,#178721,#178722,#178723,#178724,
#178725,#178726,#178727,#178728,#178729,#178730,#178731,#178732),
 .UNSPECIFIED.,.F.,.F.,(4,2,2,2,2,2,2,2,2,2,2,2,2,2,2,2,2,2,2,2,2,2,2,2,
2,2,2,2,2,2,2,2,2,2,2,2,2,2,2,2,2,4),(-11.1284471789905,-10.9816587208291,
-10.8221212812395,-10.5788393403607,-10.4617444480828,-10.2185900739436,
-10.0653161343258,-9.82206320327862,-9.61454252856661,-9.49715897724724,
-9.18835062284835,-9.06994520510295,-8.91395148058202,-8.67068666495257,
-8.55470868504613,-8.31162166341757,-8.04192503012683,-7.92357624744711,
-7.77151825007441,-7.52827892879812,-7.40712771267413,-7.16404476106431,
-6.89478333943309,-6.77645862986625,-6.62598533905963,-6.38276068494049,
-6.19286058726435,-5.97177573631606,-5.85343274268845,-5.61017529353358,
-5.49377026376138,-5.25068435595605,-5.11190848598995,-4.86883056632006,
-4.59961981470766,-4.48129985821881,-4.33099374628005,-4.0877753196181,
-3.89883471810049,-3.67904334786015,-3.56086407502634,-3.42395895046783),
 .UNSPECIFIED.);
#30251=B_SPLINE_CURVE_WITH_KNOTS('',3,(#178737,#178738,#178739,#178740,
#178741,#178742,#178743,#178744,#178745,#178746,#178747,#178748,#178749,
#178750,#178751,#178752,#178753,#178754,#178755,#178756,#178757,#178758,
#178759,#178760,#178761,#178762,#178763,#178764,#178765,#178766,#178767,
#178768,#178769,#178770,#178771,#178772,#178773,#178774,#178775,#178776,
#178777,#178778,#178779,#178780,#178781,#178782,#178783,#178784,#178785,
#178786,#178787,#178788,#178789,#178790,#178791,#178792,#178793,#178794,
#178795,#178796,#178797,#178798,#178799,#178800,#178801,#178802,#178803,
#178804,#178805,#178806,#178807,#178808,#178809,#178810,#178811,#178812,
#178813,#178814),.UNSPECIFIED.,.F.,.F.,(4,2,2,2,2,2,2,2,2,2,2,2,2,2,2,2,
2,2,2,2,2,2,2,2,2,2,2,2,2,2,2,2,2,2,2,2,2,2,4),(-19.2614576637728,-19.1356789719326,
-18.9731201279323,-18.7299508942672,-18.584783367083,-18.3416704020533,
-18.2006804311134,-17.9575847946136,-17.8177162848732,-17.5746255386636,
-17.3364643703782,-17.0110447446521,-16.893675924676,-16.6601686346933,
-16.4246089396369,-16.2865539568494,-16.0434714014953,-15.9223218853332,
-15.6790861072034,-15.439812074119,-15.2022771564619,-14.972500515759,-14.7740011427573,
-14.5307675167468,-14.3788774059206,-14.2605320044324,-13.9908835424712,
-13.74780064827,-13.5097367539058,-13.2746224555694,-13.0313626288571,-12.8556969244336,
-12.612493001893,-12.464613656871,-12.2214846886535,-12.1045468764796,-11.8612760424733,
-11.7030254218495,-11.5566456717678),.UNSPECIFIED.);
#30252=B_SPLINE_CURVE_WITH_KNOTS('',3,(#178816,#178817,#178818,#178819,
#178820,#178821,#178822,#178823,#178824,#178825,#178826,#178827,#178828,
#178829,#178830,#178831,#178832,#178833,#178834,#178835,#178836,#178837,
#178838,#178839,#178840,#178841,#178842,#178843,#178844,#178845,#178846,
#178847,#178848,#178849,#178850,#178851,#178852,#178853,#178854,#178855),
 .UNSPECIFIED.,.F.,.F.,(4,2,2,2,2,2,2,2,2,2,2,2,2,2,2,2,2,2,2,4),(-3.42395895046783,
-3.31762163229697,-3.10420599987773,-2.98677630963011,-2.74955318449751,
-2.52785333895686,-2.40944089100547,-2.16618638678871,-2.04940406440818,
-1.8063065177699,-1.66329915599726,-1.42016381120343,-1.26694861534978,
-1.02371503625448,-0.9025623522204,-0.659474909044351,-0.518219698477484,
-0.260456869351534,-0.130812079682504,-8.37234198767857E-5),
 .UNSPECIFIED.);
#30253=B_SPLINE_CURVE_WITH_KNOTS('',3,(#178856,#178857,#178858,#178859,
#178860,#178861,#178862,#178863,#178864,#178865,#178866,#178867,#178868,
#178869,#178870,#178871,#178872,#178873,#178874,#178875,#178876,#178877,
#178878,#178879,#178880,#178881,#178882,#178883,#178884,#178885,#178886,
#178887,#178888,#178889,#178890,#178891,#178892,#178893,#178894,#178895,
#178896,#178897,#178898,#178899,#178900,#178901),.UNSPECIFIED.,.F.,.F.,
(4,2,2,2,2,2,2,2,2,2,2,2,2,2,2,2,2,2,2,2,2,2,4),(-15.8354657754405,-15.6407458592451,
-15.4634984810298,-15.224746948074,-15.0754563288153,-14.9781844851558,
-14.4958306045442,-14.302961113374,-14.0985025945051,-13.8652929473164,
-13.6951623652772,-13.4855741019692,-13.2508958722351,-13.078530665073,
-12.8679347864287,-12.6329351583833,-12.4473201408781,-12.2420452632793,
-12.0880584712123,-11.9269121240055,-11.8242338140593,-11.6207006516122,
-11.5542914416033),.UNSPECIFIED.);
#30254=B_SPLINE_CURVE_WITH_KNOTS('',3,(#178907,#178908,#178909,#178910,
#178911,#178912,#178913,#178914,#178915,#178916,#178917,#178918,#178919,
#178920,#178921,#178922,#178923,#178924,#178925,#178926,#178927,#178928,
#178929,#178930,#178931,#178932,#178933,#178934,#178935,#178936,#178937,
#178938),.UNSPECIFIED.,.F.,.F.,(4,2,2,2,2,2,2,2,2,2,2,2,2,2,2,4),(-4.28434131558935,
-4.09277740390565,-3.61917123484337,-3.44763570279824,-3.18732168422942,
-2.69760137829887,-2.47655354440947,-2.23097941886294,-1.99516743825397,
-1.79887979205484,-1.30903271526569,-1.139548317617,-0.874036586908317,
-0.506625225075278,-0.275259934209563,-6.25946676274787E-5),
 .UNSPECIFIED.);
#30255=B_SPLINE_CURVE_WITH_KNOTS('',3,(#178939,#178940,#178941,#178942,
#178943,#178944,#178945,#178946,#178947,#178948,#178949,#178950,#178951,
#178952,#178953,#178954,#178955,#178956,#178957,#178958,#178959,#178960,
#178961,#178962,#178963,#178964,#178965,#178966,#178967,#178968,#178969,
#178970,#178971,#178972,#178973,#178974,#178975,#178976),.UNSPECIFIED.,
 .F.,.F.,(4,2,2,2,2,2,2,2,2,2,2,2,2,2,2,2,2,2,4),(-22.6854834825577,-22.56281589728,
-22.4409718299283,-22.2016930444766,-22.0443790072972,-21.8011428851532,
-21.6479506659735,-21.4048125035339,-21.166216579999,-20.9302791714888,
-20.7043149936291,-20.5112109918504,-20.2679881685403,-20.1500823996117,
-19.9068055479873,-19.7395638044544,-19.4963842851851,-19.3789539628455,
-19.2614576637728),.UNSPECIFIED.);
#30256=B_SPLINE_CURVE_WITH_KNOTS('',3,(#178977,#178978,#178979,#178980,
#178981,#178982,#178983,#178984,#178985,#178986,#178987,#178988,#178989,
#178990,#178991,#178992,#178993,#178994,#178995,#178996,#178997,#178998,
#178999,#179000,#179001,#179002,#179003,#179004,#179005,#179006,#179007,
#179008,#179009,#179010,#179011,#179012,#179013,#179014,#179015,#179016,
#179017,#179018,#179019,#179020,#179021,#179022,#179023,#179024,#179025,
#179026,#179027,#179028,#179029,#179030,#179031,#179032,#179033,#179034,
#179035,#179036,#179037,#179038,#179039,#179040,#179041,#179042,#179043,
#179044,#179045,#179046,#179047,#179048,#179049,#179050,#179051,#179052,
#179053,#179054,#179055,#179056,#179057,#179058,#179059,#179060),
 .UNSPECIFIED.,.F.,.F.,(4,2,2,2,2,2,2,2,2,2,2,2,2,2,2,2,2,2,2,2,2,2,2,2,
2,2,2,2,2,2,2,2,2,2,2,2,2,2,2,2,2,4),(-11.5542914416033,-11.4737373012928,
-11.309482051677,-11.12712473689,-10.8918422034198,-10.755109644318,-10.6080076524658,
-10.395068669024,-10.1594521898136,-9.97180536976226,-9.7665090044771,-9.61243658395786,
-9.45133180206899,-9.34869787814915,-9.14516201698245,-8.91245253192468,
-8.73952193900105,-8.531902825353,-8.29781529126438,-8.12528871999226,-7.9156016238263,
-7.70024882936839,-7.49762229510223,-7.18415226895485,-6.97468363629993,
-6.80124038036845,-6.56701043783358,-6.35892698651081,-6.18711460646771,
-5.95441407950802,-5.75090105180435,-5.64822728207524,-5.48708701340564,
-5.33311721246657,-5.12786052318682,-4.9400333125358,-4.70438356181232,
-4.49131096231414,-4.34481309486669,-4.20821925860371,-3.97021584717785,
-3.8512796228323),.UNSPECIFIED.);
#30257=B_SPLINE_CURVE_WITH_KNOTS('',3,(#179067,#179068,#179069,#179070,
#179071,#179072,#179073,#179074),.UNSPECIFIED.,.F.,.F.,(4,2,2,4),(-12.5667440997737,
-12.3948646496968,-12.2315921270525,-11.9950102079231),.UNSPECIFIED.);
#30258=B_SPLINE_CURVE_WITH_KNOTS('',3,(#179082,#179083,#179084,#179085,
#179086,#179087,#179088,#179089,#179090,#179091,#179092,#179093,#179094,
#179095,#179096,#179097,#179098,#179099,#179100,#179101,#179102,#179103,
#179104,#179105,#179106,#179107,#179108,#179109,#179110,#179111,#179112,
#179113,#179114,#179115,#179116,#179117,#179118,#179119,#179120,#179121,
#179122,#179123,#179124,#179125,#179126,#179127,#179128,#179129,#179130,
#179131,#179132,#179133,#179134,#179135,#179136,#179137,#179138,#179139,
#179140,#179141),.UNSPECIFIED.,.F.,.F.,(4,2,2,2,2,2,2,2,2,2,2,2,2,2,2,2,
2,2,2,2,2,2,2,2,2,2,2,2,2,4),(-11.9950102079231,-11.9174457962354,-11.7508295781321,
-11.3974253956048,-11.145701176373,-10.9105100206839,-10.6766139857417,
-10.1854286855557,-10.015992362905,-9.84730729815986,-9.50844590171839,
-9.01935539446705,-8.86994604617293,-8.62945896761266,-8.37107887868964,
-7.87982978971591,-7.69943489551864,-7.3543871731509,-7.09964540660761,
-6.78873130182666,-6.51898063956417,-6.28324949673751,-6.04828226035897,
-5.82497750860756,-5.35946271870781,-5.19008739124356,-4.91855369036197,
-4.54959355051724,-4.31459941253855,-4.28434131558935),.UNSPECIFIED.);
#30259=B_SPLINE_CURVE_WITH_KNOTS('',3,(#179143,#179144,#179145,#179146,
#179147,#179148,#179149,#179150,#179151,#179152,#179153,#179154,#179155,
#179156,#179157,#179158,#179159,#179160,#179161,#179162,#179163,#179164,
#179165,#179166,#179167,#179168,#179169,#179170,#179171,#179172,#179173,
#179174,#179175,#179176,#179177,#179178,#179179,#179180,#179181,#179182,
#179183,#179184,#179185,#179186,#179187,#179188,#179189,#179190),
 .UNSPECIFIED.,.F.,.F.,(4,2,2,2,2,2,2,2,2,2,2,2,2,2,2,2,2,2,2,2,2,2,2,4),
(-3.8512796228323,-3.7901986030621,-3.62600036533853,-3.478932106501,-3.27538901373182,
-3.17281013873208,-3.01175246892729,-2.85756470629415,-2.65224064392687,
-2.46482663385682,-2.22925087842699,-2.01648262408061,-1.86870024940216,
-1.73196153851578,-1.4991536801006,-1.3141785407599,-1.14882249401481,-1.00412990208225,
-0.801059083462348,-0.582700972005783,-0.355531059708101,-0.182241705505865,
-0.109215112418338,-9.99999998363421E-7),.UNSPECIFIED.);
#30260=B_SPLINE_CURVE_WITH_KNOTS('',3,(#179192,#179193,#179194,#179195,
#179196,#179197,#179198,#179199,#179200,#179201,#179202,#179203,#179204,
#179205,#179206,#179207,#179208,#179209),.UNSPECIFIED.,.F.,.F.,(4,2,2,2,
2,2,2,2,4),(-1.56872780698428,-1.44403063362972,-1.12597350523431,-0.975660481161639,
-0.784391357146069,-0.59140859172425,-0.401362373433348,-0.087630267916436,
-4.32669937617874E-5),.UNSPECIFIED.);
#30261=B_SPLINE_CURVE_WITH_KNOTS('',3,(#179212,#179213,#179214,#179215,
#179216,#179217,#179218,#179219,#179220,#179221,#179222,#179223,#179224,
#179225,#179226,#179227,#179228,#179229,#179230,#179231,#179232,#179233,
#179234,#179235,#179236,#179237,#179238,#179239,#179240,#179241,#179242,
#179243,#179244,#179245,#179246,#179247,#179248,#179249,#179250,#179251,
#179252,#179253,#179254,#179255,#179256,#179257,#179258,#179259,#179260,
#179261,#179262,#179263,#179264,#179265,#179266,#179267,#179268,#179269,
#179270,#179271,#179272,#179273,#179274,#179275,#179276,#179277,#179278,
#179279,#179280,#179281,#179282,#179283,#179284,#179285,#179286,#179287,
#179288,#179289,#179290,#179291),.UNSPECIFIED.,.F.,.F.,(4,2,2,2,2,2,2,2,
2,2,2,2,2,2,2,2,2,2,2,2,2,2,2,2,2,2,2,2,2,2,2,2,2,2,2,2,2,2,2,4),(1.00000000916034E-6,
0.213754930701631,0.424652319564036,0.565040153296804,0.748075759262127,
1.05142999748217,1.25223264793173,1.50715507366388,1.76061269237607,2.01941808507526,
2.26964944794214,2.47651392626711,2.73003327533967,2.98431110662871,3.24346008377567,
3.50188237345356,3.6267924102787,3.8729079603262,4.08710371160095,4.28624559950554,
4.41150404599036,4.68071417586692,4.89967370396659,5.07419479348004,5.29610569553035,
5.47890193858856,5.70169182511378,5.91354244510472,6.13506182294941,6.26094691361958,
6.51995060806452,6.73927748471563,6.96718021692218,7.11944389614993,7.3777879311047,
7.50229063002226,7.76088809123817,7.96057223441664,8.08559790968841,8.20599054997932),
 .UNSPECIFIED.);
#30262=B_SPLINE_CURVE_WITH_KNOTS('',3,(#179292,#179293,#179294,#179295,
#179296,#179297,#179298,#179299,#179300,#179301,#179302,#179303,#179304,
#179305,#179306,#179307,#179308,#179309,#179310,#179311,#179312,#179313,
#179314,#179315,#179316,#179317,#179318,#179319,#179320,#179321,#179322,
#179323,#179324,#179325,#179326,#179327,#179328,#179329,#179330,#179331,
#179332,#179333,#179334,#179335,#179336,#179337,#179338,#179339,#179340,
#179341,#179342,#179343,#179344,#179345,#179346,#179347,#179348,#179349,
#179350,#179351,#179352,#179353,#179354,#179355,#179356,#179357,#179358,
#179359,#179360,#179361,#179362,#179363,#179364,#179365,#179366,#179367,
#179368,#179369,#179370,#179371,#179372,#179373),.UNSPECIFIED.,.F.,.F.,
(4,2,2,2,2,2,2,2,2,2,2,2,2,2,2,2,2,2,2,2,2,2,2,2,2,2,2,2,2,2,2,2,2,2,2,
2,2,2,2,2,4),(15.9563811041735,15.9737975928771,16.188144625583,16.4403174813183,
16.6990099245498,16.9507148240286,17.2074066749168,17.4259263304847,17.6367507053452,
17.8957326470844,18.0212038054511,18.2460623414005,18.436300514819,18.6585432543082,
18.8698740658398,19.0932433887016,19.286315914036,19.5142197774173,19.6388520817395,
19.8986455059131,20.0628063040985,20.2809247137134,20.4746673369814,20.6873209945832,
20.8803418454722,21.0898020808175,21.2889726415437,21.4941317239042,21.7182599168424,
21.9192434783725,22.173550582982,22.2982001664574,22.5570948821,22.8158110382015,
22.9431610993941,23.1412950840882,23.3935731392472,23.5807736260057,23.724556486473,
23.9421164922607,24.1619673706865),.UNSPECIFIED.);
#30263=B_SPLINE_CURVE_WITH_KNOTS('',3,(#179377,#179378,#179379,#179380,
#179381,#179382,#179383,#179384,#179385,#179386,#179387,#179388,#179389,
#179390,#179391,#179392),.UNSPECIFIED.,.F.,.F.,(4,2,2,2,2,2,2,4),(-5.3403698058518,
-5.10302024972618,-4.85331064876673,-4.3722544378929,-3.88453013965518,
-3.63186010165686,-3.38655743613479,-3.33078402932654),.UNSPECIFIED.);
#30264=B_SPLINE_CURVE_WITH_KNOTS('',3,(#179396,#179397,#179398,#179399,
#179400,#179401,#179402,#179403,#179404,#179405,#179406,#179407,#179408,
#179409,#179410,#179411,#179412,#179413,#179414,#179415,#179416,#179417),
 .UNSPECIFIED.,.F.,.F.,(4,2,2,2,2,2,2,2,2,2,4),(-3.33078402932654,-3.14577878108155,
-2.6696933689128,-2.42517438026941,-2.18777430397266,-1.69235110044299,
-1.45012215009031,-1.21210349138623,-0.975414798478184,-0.488398210557989,
-4.75981067121614E-5),.UNSPECIFIED.);
#30265=B_SPLINE_CURVE_WITH_KNOTS('',3,(#179419,#179420,#179421,#179422,
#179423,#179424,#179425,#179426,#179427,#179428,#179429,#179430,#179431,
#179432,#179433,#179434,#179435,#179436,#179437,#179438,#179439,#179440,
#179441,#179442,#179443,#179444,#179445,#179446,#179447,#179448,#179449,
#179450,#179451,#179452,#179453,#179454,#179455,#179456,#179457,#179458,
#179459,#179460,#179461,#179462,#179463,#179464,#179465,#179466,#179467,
#179468,#179469,#179470,#179471,#179472,#179473,#179474,#179475,#179476,
#179477,#179478,#179479,#179480,#179481,#179482,#179483,#179484,#179485),
 .UNSPECIFIED.,.F.,.F.,(4,3,3,3,3,3,3,3,3,3,3,3,3,3,3,3,3,3,3,3,3,3,4),
(0.,0.0532797188796114,0.106117363864123,0.125,0.176897081798127,0.229324525544369,
0.25,0.301861332022725,0.353569755832101,0.405192326669166,0.456691995603618,
0.499999999999999,0.551296718367494,0.602946326486467,0.654794611099575,
0.706987743443309,0.749999999999998,0.803309497918933,0.856238158518513,
0.874999999999999,0.929869764525177,0.984191399200626,0.999999665677158),
 .UNSPECIFIED.);
#30266=B_SPLINE_CURVE_WITH_KNOTS('',3,(#179487,#179488,#179489,#179490,
#179491,#179492,#179493,#179494,#179495,#179496),.UNSPECIFIED.,.F.,.F.,
(4,2,2,2,4),(-1.36676107014535,-1.02924695186405,-0.680886324591822,-0.34453153614729,
-6.48039110316922E-5),.UNSPECIFIED.);
#30267=B_SPLINE_CURVE_WITH_KNOTS('',3,(#179497,#179498,#179499,#179500),
 .UNSPECIFIED.,.F.,.F.,(4,4),(-0.000734763449235485,0.),.UNSPECIFIED.);
#30268=B_SPLINE_CURVE_WITH_KNOTS('',3,(#179750,#179751,#179752,#179753,
#179754,#179755,#179756,#179757,#179758,#179759,#179760,#179761,#179762,
#179763,#179764,#179765,#179766,#179767,#179768,#179769,#179770,#179771,
#179772,#179773,#179774,#179775,#179776,#179777,#179778,#179779,#179780,
#179781,#179782,#179783,#179784,#179785,#179786,#179787,#179788,#179789,
#179790,#179791,#179792,#179793,#179794,#179795,#179796,#179797,#179798,
#179799,#179800,#179801,#179802,#179803,#179804,#179805,#179806,#179807,
#179808,#179809,#179810,#179811,#179812,#179813,#179814,#179815,#179816,
#179817,#179818,#179819,#179820,#179821,#179822,#179823,#179824,#179825,
#179826,#179827,#179828,#179829,#179830,#179831,#179832,#179833,#179834,
#179835,#179836,#179837,#179838,#179839,#179840,#179841,#179842,#179843,
#179844,#179845,#179846,#179847,#179848,#179849,#179850,#179851,#179852,
#179853,#179854,#179855,#179856,#179857,#179858,#179859,#179860,#179861,
#179862,#179863,#179864,#179865,#179866,#179867,#179868,#179869,#179870,
#179871,#179872,#179873,#179874,#179875,#179876,#179877,#179878,#179879,
#179880,#179881,#179882,#179883,#179884,#179885,#179886,#179887,#179888,
#179889,#179890,#179891,#179892,#179893,#179894,#179895,#179896,#179897,
#179898,#179899,#179900,#179901,#179902,#179903,#179904,#179905,#179906,
#179907,#179908,#179909,#179910,#179911,#179912,#179913,#179914,#179915,
#179916,#179917,#179918,#179919,#179920,#179921,#179922,#179923,#179924,
#179925,#179926,#179927,#179928,#179929,#179930,#179931,#179932,#179933,
#179934,#179935,#179936,#179937,#179938,#179939,#179940,#179941,#179942,
#179943,#179944,#179945,#179946,#179947,#179948,#179949,#179950,#179951,
#179952,#179953,#179954,#179955,#179956,#179957,#179958,#179959,#179960,
#179961,#179962,#179963,#179964,#179965,#179966,#179967,#179968,#179969,
#179970,#179971,#179972,#179973,#179974,#179975,#179976,#179977,#179978,
#179979,#179980,#179981,#179982,#179983,#179984,#179985,#179986,#179987,
#179988,#179989,#179990,#179991,#179992,#179993,#179994,#179995,#179996,
#179997,#179998,#179999,#180000,#180001,#180002,#180003,#180004,#180005,
#180006,#180007,#180008,#180009,#180010,#180011,#180012,#180013,#180014,
#180015),.UNSPECIFIED.,.F.,.F.,(4,2,2,2,2,2,2,2,2,2,2,2,2,2,2,2,2,2,2,2,
2,2,2,2,2,2,2,2,2,2,2,2,2,2,2,2,2,2,2,2,2,2,2,2,2,2,2,2,2,2,2,2,2,2,2,2,
2,2,2,2,2,2,2,2,2,2,2,2,2,2,2,2,2,2,2,2,2,2,2,2,2,2,2,2,2,2,2,2,2,2,2,2,
2,2,2,2,2,2,2,2,2,2,2,2,2,2,2,2,2,2,2,2,2,2,2,2,2,2,2,2,2,2,2,2,2,2,2,2,
2,2,2,2,4),(0.00790828593611698,0.135265930291889,0.267467597358619,0.533750940167357,
0.88017574947923,1.13384054666904,1.41070844498502,1.59304811912023,1.75172514557715,
1.94683197777222,2.11230898000431,2.2183789781365,2.42776377877795,2.62555120627117,
2.76879848422111,2.84874922368211,2.95782682962964,3.14207307762776,3.25663406363165,
3.37303424343138,3.45626456111032,3.52892374114935,3.6857389432425,3.80006939109491,
3.88555748851367,4.03204550791092,4.10568247069694,4.17075352363226,4.33697990742952,
4.47525429526118,4.54231004104649,4.69175162177885,4.75810401002136,4.81934676172847,
4.98088188776317,5.06503890354536,5.1321151904307,5.30211693017162,5.38412488189451,
5.44913617798401,5.62479169811705,5.69791337660177,5.76286233196133,5.91136026020286,
6.04925408777556,6.11298181775794,6.23610551115398,6.31388054876702,6.38380024863477,
6.5432048593396,6.65174213941674,6.73361681103904,6.84908481495156,6.96566430926586,
7.06231774977973,7.25739291090475,7.36935564096079,7.49481348313,7.61574875549503,
7.85194025684748,7.97321502503676,8.08120256050554,8.19960850771165,8.51294062655963,
8.65864759138126,8.89994724302448,9.15209692020237,9.39092942283465,9.8907051436538,
10.1408102616569,10.5878990435705,10.6957027295127,10.9247285148082,11.1721695044457,
11.3026464814219,11.4127050574303,11.5387697472141,11.7749710961387,11.8944602329429,
12.0206170420862,12.1515274285258,12.3960230599727,12.488159385815,12.6185402384999,
12.6893810027722,12.8337840499673,13.0004068655612,13.0719250791122,13.1514270639328,
13.2900322788783,13.360499232878,13.4504930252814,13.6181564670971,13.6835742421503,
13.7534366573758,13.9354223495435,14.0011227284056,14.0851924898259,14.2451036661492,
14.3093382614856,14.3835463997154,14.5778804557065,14.6416178904133,14.7210686769463,
14.8716856282844,14.940114896237,15.0236871260087,15.2210857305321,15.2872921270163,
15.3680758518447,15.5054362572902,15.590558560566,15.7067094494271,15.8567404575721,
15.9290430710459,16.035996173057,16.1380191692964,16.2541464373657,16.4511595599156,
16.5500800259854,16.6242233687588,16.6963137053059,16.8009540412491,16.9203081431285,
17.1808011324626,17.282359025085,17.4399399592422,17.6184937765128,17.8672726158994,
17.9911861104215,18.2371444098655,18.5095375574028,18.789319718825),
 .UNSPECIFIED.);
#30269=B_SPLINE_CURVE_WITH_KNOTS('',3,(#180157,#180158,#180159,#180160,
#180161,#180162,#180163,#180164,#180165,#180166,#180167,#180168,#180169,
#180170,#180171,#180172,#180173,#180174,#180175,#180176,#180177,#180178,
#180179,#180180,#180181,#180182,#180183,#180184,#180185,#180186,#180187,
#180188,#180189,#180190,#180191,#180192,#180193,#180194,#180195,#180196,
#180197,#180198,#180199,#180200,#180201,#180202,#180203,#180204,#180205,
#180206,#180207,#180208,#180209,#180210,#180211,#180212,#180213,#180214,
#180215,#180216,#180217,#180218,#180219,#180220,#180221,#180222,#180223,
#180224,#180225,#180226,#180227,#180228,#180229,#180230,#180231,#180232,
#180233,#180234,#180235,#180236,#180237,#180238),.UNSPECIFIED.,.F.,.F.,
(4,2,2,2,2,2,2,2,2,2,2,2,2,2,2,2,2,2,2,2,2,2,2,2,2,2,2,2,2,2,2,2,2,2,2,
2,2,2,2,2,4),(-14.2732703758709,-13.8912273375201,-13.6142499111422,-13.3975932236668,
-13.1227155431991,-12.7070233843363,-12.382403721312,-12.1293949735596,
-11.8703642014538,-11.535385037698,-11.1414389160712,-10.8461410004354,
-10.5760851451155,-10.229212584883,-9.73704557040598,-9.39335342116224,
-9.12378600302777,-8.81489519474117,-8.39716574472202,-8.04541518662001,
-7.77721020461666,-7.50917494410743,-7.15370825665347,-6.694616193426,-6.35436303692717,
-6.06376512693916,-5.68296158713199,-5.09892163723771,-4.68369409175826,
-4.35935666716764,-4.01204603446286,-3.53687730816414,-3.0882622443312,
-2.75857559247952,-2.45520533882133,-2.06641699455647,-1.51781117593839,
-1.13911402161754,-0.846466340153964,-0.481778164862173,-7.79037809220391E-5),
 .UNSPECIFIED.);
#30270=B_SPLINE_CURVE_WITH_KNOTS('',3,(#180507,#180508,#180509,#180510,
#180511,#180512),.UNSPECIFIED.,.F.,.F.,(4,2,4),(-0.0902565102820884,-0.0451906624768086,
-0.000194550672140855),.UNSPECIFIED.);
#30271=B_SPLINE_CURVE_WITH_KNOTS('',3,(#180534,#180535,#180536,#180537,
#180538,#180539,#180540,#180541,#180542,#180543,#180544,#180545,#180546,
#180547,#180548,#180549,#180550,#180551,#180552,#180553,#180554,#180555,
#180556,#180557,#180558,#180559,#180560,#180561,#180562,#180563,#180564,
#180565,#180566,#180567,#180568,#180569,#180570,#180571,#180572,#180573,
#180574,#180575,#180576,#180577,#180578,#180579,#180580,#180581,#180582,
#180583,#180584,#180585,#180586,#180587,#180588,#180589,#180590,#180591),
 .UNSPECIFIED.,.F.,.F.,(4,3,3,3,3,3,3,3,3,3,3,3,3,3,3,3,3,3,3,4),(-1.28896142244996,
-1.09309231306789,-1.04016081898117,-0.980183490937908,-0.885023600722137,
-0.791562904177703,-0.670254571147595,-0.644748735286477,-0.63409310387645,
-0.626279232155984,-0.469588976339915,-0.352102611119142,-0.310009489205054,
-0.249406568724682,-0.188707985000504,-0.175752395276352,-0.142257802210724,
-0.0813352071390198,-0.0211767799124928,-1.50340975617814E-6),
 .UNSPECIFIED.);
#30272=B_SPLINE_CURVE_WITH_KNOTS('',3,(#180616,#180617,#180618,#180619,
#180620,#180621,#180622,#180623,#180624,#180625,#180626,#180627,#180628,
#180629,#180630,#180631,#180632,#180633,#180634,#180635,#180636,#180637,
#180638,#180639,#180640,#180641,#180642,#180643,#180644,#180645,#180646,
#180647,#180648,#180649,#180650,#180651,#180652,#180653,#180654,#180655,
#180656,#180657,#180658,#180659,#180660,#180661,#180662,#180663,#180664,
#180665,#180666,#180667,#180668,#180669,#180670,#180671,#180672,#180673),
 .UNSPECIFIED.,.F.,.F.,(4,3,3,3,3,3,3,3,3,3,3,3,3,3,3,3,3,3,3,4),(0.000196331256314133,
0.195854367371089,0.245817836587428,0.308742496769599,0.403496982746037,
0.491306783782198,0.608890768221054,0.644062191156574,0.654689003663857,
0.65473511082066,0.81371042122958,0.932829188307031,0.979410739452192,1.03972898457711,
1.10013481239701,1.11172797209075,1.14748205288075,1.20898204679883,1.26971077107247,
1.29001475424187),.UNSPECIFIED.);
#30273=B_SPLINE_CURVE_WITH_KNOTS('',3,(#180694,#180695,#180696,#180697,
#180698,#180699),.UNSPECIFIED.,.F.,.F.,(4,2,4),(-0.0900560308119693,-0.0451018328691558,
-1.01924371514621E-5),.UNSPECIFIED.);
#31315=CIRCLE('',#80801,12.25);
#31316=CIRCLE('',#80806,12.25);
#31317=CIRCLE('',#80808,10.5);
#31318=CIRCLE('',#80809,10.5);
#31319=CIRCLE('',#80811,12.25);
#31320=CIRCLE('',#80814,13.25000025523);
#31321=CIRCLE('',#80816,16.);
#31322=CIRCLE('',#80817,16.);
#31323=CIRCLE('',#80818,16.);
#31324=CIRCLE('',#80819,16.);
#31325=CIRCLE('',#80820,16.);
#31326=CIRCLE('',#80821,14.);
#31327=CIRCLE('',#80822,16.);
#31328=CIRCLE('',#80823,16.);
#31329=CIRCLE('',#80825,16.);
#31330=CIRCLE('',#80826,16.);
#31331=CIRCLE('',#80827,16.);
#31332=CIRCLE('',#80828,16.);
#31333=CIRCLE('',#80829,16.);
#31334=CIRCLE('',#80830,14.);
#31335=CIRCLE('',#80831,16.);
#31336=CIRCLE('',#80832,16.);
#34872=VERTEX_POINT('',#177997);
#34873=VERTEX_POINT('',#177998);
#34874=VERTEX_POINT('',#178000);
#34875=VERTEX_POINT('',#178043);
#34876=VERTEX_POINT('',#178078);
#34877=VERTEX_POINT('',#178153);
#34878=VERTEX_POINT('',#178154);
#34879=VERTEX_POINT('',#178319);
#34880=VERTEX_POINT('',#178320);
#34881=VERTEX_POINT('',#178322);
#34882=VERTEX_POINT('',#178333);
#34883=VERTEX_POINT('',#178349);
#34884=VERTEX_POINT('',#178350);
#34885=VERTEX_POINT('',#178352);
#34886=VERTEX_POINT('',#178397);
#34887=VERTEX_POINT('',#178408);
#34888=VERTEX_POINT('',#178419);
#34889=VERTEX_POINT('',#178421);
#34890=VERTEX_POINT('',#178432);
#34891=VERTEX_POINT('',#178443);
#34892=VERTEX_POINT('',#178486);
#34893=VERTEX_POINT('',#178568);
#34894=VERTEX_POINT('',#178569);
#34895=VERTEX_POINT('',#178734);
#34896=VERTEX_POINT('',#178735);
#34897=VERTEX_POINT('',#178815);
#34898=VERTEX_POINT('',#178903);
#34899=VERTEX_POINT('',#178904);
#34900=VERTEX_POINT('',#178906);
#34901=VERTEX_POINT('',#179062);
#34902=VERTEX_POINT('',#179063);
#34903=VERTEX_POINT('',#179065);
#34904=VERTEX_POINT('',#179076);
#34905=VERTEX_POINT('',#179078);
#34906=VERTEX_POINT('',#179142);
#34907=VERTEX_POINT('',#179191);
#34908=VERTEX_POINT('',#179375);
#34909=VERTEX_POINT('',#179376);
#34910=VERTEX_POINT('',#179393);
#34911=VERTEX_POINT('',#179418);
#34912=VERTEX_POINT('',#179486);
#34913=VERTEX_POINT('',#179502);
#34914=VERTEX_POINT('',#179503);
#34915=VERTEX_POINT('',#179507);
#34916=VERTEX_POINT('',#179509);
#34917=VERTEX_POINT('',#179513);
#34918=VERTEX_POINT('',#179515);
#34919=VERTEX_POINT('',#179519);
#34920=VERTEX_POINT('',#179521);
#34921=VERTEX_POINT('',#179525);
#34922=VERTEX_POINT('',#179527);
#34923=VERTEX_POINT('',#179531);
#34924=VERTEX_POINT('',#179533);
#34925=VERTEX_POINT('',#179536);
#34926=VERTEX_POINT('',#179538);
#34927=VERTEX_POINT('',#179544);
#34928=VERTEX_POINT('',#179545);
#34929=VERTEX_POINT('',#179549);
#34930=VERTEX_POINT('',#179551);
#34931=VERTEX_POINT('',#179555);
#34932=VERTEX_POINT('',#179557);
#34933=VERTEX_POINT('',#179561);
#34934=VERTEX_POINT('',#179563);
#34935=VERTEX_POINT('',#179567);
#34936=VERTEX_POINT('',#179569);
#34937=VERTEX_POINT('',#179573);
#34938=VERTEX_POINT('',#179575);
#34939=VERTEX_POINT('',#179578);
#34940=VERTEX_POINT('',#179580);
#43181=EDGE_CURVE('',#34872,#34873,#3159,.T.);
#43182=EDGE_CURVE('',#34874,#34873,#30234,.F.);
#43183=EDGE_CURVE('',#34875,#34874,#30235,.T.);
#43184=EDGE_CURVE('',#34876,#34875,#3160,.T.);
#43185=EDGE_CURVE('',#34876,#34872,#30236,.T.);
#43186=EDGE_CURVE('',#34877,#34878,#3161,.T.);
#43187=EDGE_CURVE('',#34873,#34878,#30237,.F.);
#43188=EDGE_CURVE('',#34872,#34877,#30238,.T.);
#43189=EDGE_CURVE('',#34879,#34880,#3162,.T.);
#43190=EDGE_CURVE('',#34879,#34881,#30239,.T.);
#43191=EDGE_CURVE('',#34881,#34882,#30240,.T.);
#43192=EDGE_CURVE('',#34880,#34882,#30241,.T.);
#43193=EDGE_CURVE('',#34883,#34884,#3163,.T.);
#43194=EDGE_CURVE('',#34884,#34885,#30242,.T.);
#43195=EDGE_CURVE('',#34885,#34886,#30243,.T.);
#43196=EDGE_CURVE('',#34886,#34887,#30244,.T.);
#43197=EDGE_CURVE('',#34887,#34888,#3164,.T.);
#43198=EDGE_CURVE('',#34888,#34889,#30245,.T.);
#43199=EDGE_CURVE('',#34889,#34890,#30246,.T.);
#43200=EDGE_CURVE('',#34890,#34891,#30247,.T.);
#43201=EDGE_CURVE('',#34891,#34892,#3165,.T.);
#43202=EDGE_CURVE('',#34892,#34892,#31315,.T.);
#43203=EDGE_CURVE('',#34891,#34883,#30248,.T.);
#43204=EDGE_CURVE('',#34893,#34894,#3166,.T.);
#43205=EDGE_CURVE('',#34894,#34884,#30249,.T.);
#43206=EDGE_CURVE('',#34883,#34893,#30250,.T.);
#43207=EDGE_CURVE('',#34895,#34896,#3167,.T.);
#43208=EDGE_CURVE('',#34896,#34894,#30251,.T.);
#43209=EDGE_CURVE('',#34893,#34897,#30252,.T.);
#43210=EDGE_CURVE('',#34897,#34895,#30253,.T.);
#43211=EDGE_CURVE('',#34898,#34899,#3168,.T.);
#43212=EDGE_CURVE('',#34900,#34899,#30254,.F.);
#43213=EDGE_CURVE('',#34900,#34896,#30255,.T.);
#43214=EDGE_CURVE('',#34895,#34898,#30256,.T.);
#43215=EDGE_CURVE('',#34901,#34902,#3169,.T.);
#43216=EDGE_CURVE('',#34901,#34903,#31316,.T.);
#43217=EDGE_CURVE('',#34902,#34903,#30257,.F.);
#43218=EDGE_CURVE('',#34904,#34904,#31317,.T.);
#43219=EDGE_CURVE('',#34904,#34905,#3170,.T.);
#43220=EDGE_CURVE('',#34905,#34905,#31318,.T.);
#43221=EDGE_CURVE('',#34899,#34902,#30258,.F.);
#43222=EDGE_CURVE('',#34898,#34906,#30259,.T.);
#43223=EDGE_CURVE('',#34906,#34907,#30260,.T.);
#43224=EDGE_CURVE('',#34907,#34901,#31319,.T.);
#43225=EDGE_CURVE('',#34878,#34880,#30261,.F.);
#43226=EDGE_CURVE('',#34877,#34879,#30262,.T.);
#43227=EDGE_CURVE('',#34908,#34909,#30263,.T.);
#43228=EDGE_CURVE('',#34909,#34910,#3171,.T.);
#43229=EDGE_CURVE('',#34910,#34910,#31320,.T.);
#43230=EDGE_CURVE('',#34909,#34903,#30264,.T.);
#43231=EDGE_CURVE('',#34911,#34907,#30265,.T.);
#43232=EDGE_CURVE('',#34911,#34912,#30266,.T.);
#43233=EDGE_CURVE('',#34912,#34908,#30267,.T.);
#43234=EDGE_CURVE('',#34913,#34914,#1788,.T.);
#43235=EDGE_CURVE('',#34913,#34915,#31321,.T.);
#43236=EDGE_CURVE('',#34916,#34915,#1789,.T.);
#43237=EDGE_CURVE('',#34916,#34917,#31322,.T.);
#43238=EDGE_CURVE('',#34918,#34917,#1790,.T.);
#43239=EDGE_CURVE('',#34918,#34919,#31323,.T.);
#43240=EDGE_CURVE('',#34920,#34919,#1791,.F.);
#43241=EDGE_CURVE('',#34921,#34920,#31324,.T.);
#43242=EDGE_CURVE('',#34922,#34921,#1792,.T.);
#43243=EDGE_CURVE('',#34923,#34922,#31325,.T.);
#43244=EDGE_CURVE('',#34923,#34924,#3172,.T.);
#43245=EDGE_CURVE('',#34924,#34924,#31326,.T.);
#43246=EDGE_CURVE('',#34925,#34923,#31327,.T.);
#43247=EDGE_CURVE('',#34926,#34925,#1793,.T.);
#43248=EDGE_CURVE('',#34914,#34926,#31328,.T.);
#43249=EDGE_CURVE('',#34927,#34928,#1794,.F.);
#43250=EDGE_CURVE('',#34928,#34929,#31329,.T.);
#43251=EDGE_CURVE('',#34929,#34930,#1795,.T.);
#43252=EDGE_CURVE('',#34930,#34931,#31330,.T.);
#43253=EDGE_CURVE('',#34931,#34932,#1796,.T.);
#43254=EDGE_CURVE('',#34932,#34933,#31331,.T.);
#43255=EDGE_CURVE('',#34933,#34934,#1797,.T.);
#43256=EDGE_CURVE('',#34935,#34934,#31332,.T.);
#43257=EDGE_CURVE('',#34935,#34936,#1798,.T.);
#43258=EDGE_CURVE('',#34937,#34936,#31333,.T.);
#43259=EDGE_CURVE('',#34937,#34938,#3173,.T.);
#43260=EDGE_CURVE('',#34938,#34938,#31334,.T.);
#43261=EDGE_CURVE('',#34939,#34937,#31335,.T.);
#43262=EDGE_CURVE('',#34939,#34940,#1799,.T.);
#43263=EDGE_CURVE('',#34927,#34940,#31336,.T.);
#43264=EDGE_CURVE('',#34916,#34939,#3174,.T.);
#43265=EDGE_CURVE('',#34917,#34936,#3175,.T.);
#43266=EDGE_CURVE('',#34925,#34930,#3176,.T.);
#43267=EDGE_CURVE('',#34926,#34929,#3177,.T.);
#43268=EDGE_CURVE('',#34918,#34935,#3178,.T.);
#43269=EDGE_CURVE('',#34915,#34940,#3179,.T.);
#43270=EDGE_CURVE('',#34919,#34934,#3180,.T.);
#43271=EDGE_CURVE('',#34913,#34927,#3181,.T.);
#43272=EDGE_CURVE('',#34914,#34928,#3182,.T.);
#43273=EDGE_CURVE('',#34921,#34932,#3183,.T.);
#43274=EDGE_CURVE('',#34922,#34931,#3184,.T.);
#43275=EDGE_CURVE('',#34920,#34933,#3185,.T.);
#43276=EDGE_CURVE('',#34908,#34875,#30268,.T.);
#43277=EDGE_CURVE('',#34875,#34900,#3186,.T.);
#43278=EDGE_CURVE('',#34911,#34876,#30269,.T.);
#43279=EDGE_CURVE('',#34889,#34881,#30270,.T.);
#43280=EDGE_CURVE('',#34897,#34876,#3187,.T.);
#43281=EDGE_CURVE('',#34881,#34888,#30271,.T.);
#43282=EDGE_CURVE('',#34882,#34887,#30272,.T.);
#43283=EDGE_CURVE('',#34882,#34886,#30273,.T.);
#56697=ORIENTED_EDGE('',*,*,#43181,.T.);
#56698=ORIENTED_EDGE('',*,*,#43182,.F.);
#56699=ORIENTED_EDGE('',*,*,#43183,.F.);
#56700=ORIENTED_EDGE('',*,*,#43184,.F.);
#56701=ORIENTED_EDGE('',*,*,#43185,.T.);
#56702=ORIENTED_EDGE('',*,*,#43186,.T.);
#56703=ORIENTED_EDGE('',*,*,#43187,.F.);
#56704=ORIENTED_EDGE('',*,*,#43181,.F.);
#56705=ORIENTED_EDGE('',*,*,#43188,.T.);
#56706=ORIENTED_EDGE('',*,*,#43189,.F.);
#56707=ORIENTED_EDGE('',*,*,#43190,.T.);
#56708=ORIENTED_EDGE('',*,*,#43191,.T.);
#56709=ORIENTED_EDGE('',*,*,#43192,.F.);
#56710=ORIENTED_EDGE('',*,*,#43193,.T.);
#56711=ORIENTED_EDGE('',*,*,#43194,.T.);
#56712=ORIENTED_EDGE('',*,*,#43195,.T.);
#56713=ORIENTED_EDGE('',*,*,#43196,.T.);
#56714=ORIENTED_EDGE('',*,*,#43197,.T.);
#56715=ORIENTED_EDGE('',*,*,#43198,.T.);
#56716=ORIENTED_EDGE('',*,*,#43199,.T.);
#56717=ORIENTED_EDGE('',*,*,#43200,.T.);
#56718=ORIENTED_EDGE('',*,*,#43201,.T.);
#56719=ORIENTED_EDGE('',*,*,#43202,.F.);
#56720=ORIENTED_EDGE('',*,*,#43201,.F.);
#56721=ORIENTED_EDGE('',*,*,#43203,.T.);
#56722=ORIENTED_EDGE('',*,*,#43204,.T.);
#56723=ORIENTED_EDGE('',*,*,#43205,.T.);
#56724=ORIENTED_EDGE('',*,*,#43193,.F.);
#56725=ORIENTED_EDGE('',*,*,#43206,.T.);
#56726=ORIENTED_EDGE('',*,*,#43207,.T.);
#56727=ORIENTED_EDGE('',*,*,#43208,.T.);
#56728=ORIENTED_EDGE('',*,*,#43204,.F.);
#56729=ORIENTED_EDGE('',*,*,#43209,.T.);
#56730=ORIENTED_EDGE('',*,*,#43210,.T.);
#56731=ORIENTED_EDGE('',*,*,#43211,.T.);
#56732=ORIENTED_EDGE('',*,*,#43212,.F.);
#56733=ORIENTED_EDGE('',*,*,#43213,.T.);
#56734=ORIENTED_EDGE('',*,*,#43207,.F.);
#56735=ORIENTED_EDGE('',*,*,#43214,.T.);
#56736=ORIENTED_EDGE('',*,*,#43215,.F.);
#56737=ORIENTED_EDGE('',*,*,#43216,.T.);
#56738=ORIENTED_EDGE('',*,*,#43217,.F.);
#56739=ORIENTED_EDGE('',*,*,#43218,.T.);
#56740=ORIENTED_EDGE('',*,*,#43219,.T.);
#56741=ORIENTED_EDGE('',*,*,#43220,.T.);
#56742=ORIENTED_EDGE('',*,*,#43219,.F.);
#56743=ORIENTED_EDGE('',*,*,#43215,.T.);
#56744=ORIENTED_EDGE('',*,*,#43221,.F.);
#56745=ORIENTED_EDGE('',*,*,#43211,.F.);
#56746=ORIENTED_EDGE('',*,*,#43222,.T.);
#56747=ORIENTED_EDGE('',*,*,#43223,.T.);
#56748=ORIENTED_EDGE('',*,*,#43224,.T.);
#56749=ORIENTED_EDGE('',*,*,#43189,.T.);
#56750=ORIENTED_EDGE('',*,*,#43225,.F.);
#56751=ORIENTED_EDGE('',*,*,#43186,.F.);
#56752=ORIENTED_EDGE('',*,*,#43226,.T.);
#56753=ORIENTED_EDGE('',*,*,#43227,.T.);
#56754=ORIENTED_EDGE('',*,*,#43228,.T.);
#56755=ORIENTED_EDGE('',*,*,#43229,.F.);
#56756=ORIENTED_EDGE('',*,*,#43228,.F.);
#56757=ORIENTED_EDGE('',*,*,#43230,.T.);
#56758=ORIENTED_EDGE('',*,*,#43216,.F.);
#56759=ORIENTED_EDGE('',*,*,#43224,.F.);
#56760=ORIENTED_EDGE('',*,*,#43231,.F.);
#56761=ORIENTED_EDGE('',*,*,#43232,.T.);
#56762=ORIENTED_EDGE('',*,*,#43233,.T.);
#56763=ORIENTED_EDGE('',*,*,#43234,.F.);
#56764=ORIENTED_EDGE('',*,*,#43235,.T.);
#56765=ORIENTED_EDGE('',*,*,#43236,.F.);
#56766=ORIENTED_EDGE('',*,*,#43237,.T.);
#56767=ORIENTED_EDGE('',*,*,#43238,.F.);
#56768=ORIENTED_EDGE('',*,*,#43239,.T.);
#56769=ORIENTED_EDGE('',*,*,#43240,.F.);
#56770=ORIENTED_EDGE('',*,*,#43241,.F.);
#56771=ORIENTED_EDGE('',*,*,#43242,.F.);
#56772=ORIENTED_EDGE('',*,*,#43243,.F.);
#56773=ORIENTED_EDGE('',*,*,#43244,.T.);
#56774=ORIENTED_EDGE('',*,*,#43245,.T.);
#56775=ORIENTED_EDGE('',*,*,#43244,.F.);
#56776=ORIENTED_EDGE('',*,*,#43246,.F.);
#56777=ORIENTED_EDGE('',*,*,#43247,.F.);
#56778=ORIENTED_EDGE('',*,*,#43248,.F.);
#56779=ORIENTED_EDGE('',*,*,#43249,.T.);
#56780=ORIENTED_EDGE('',*,*,#43250,.T.);
#56781=ORIENTED_EDGE('',*,*,#43251,.T.);
#56782=ORIENTED_EDGE('',*,*,#43252,.T.);
#56783=ORIENTED_EDGE('',*,*,#43253,.T.);
#56784=ORIENTED_EDGE('',*,*,#43254,.T.);
#56785=ORIENTED_EDGE('',*,*,#43255,.T.);
#56786=ORIENTED_EDGE('',*,*,#43256,.F.);
#56787=ORIENTED_EDGE('',*,*,#43257,.T.);
#56788=ORIENTED_EDGE('',*,*,#43258,.F.);
#56789=ORIENTED_EDGE('',*,*,#43259,.T.);
#56790=ORIENTED_EDGE('',*,*,#43260,.F.);
#56791=ORIENTED_EDGE('',*,*,#43259,.F.);
#56792=ORIENTED_EDGE('',*,*,#43261,.F.);
#56793=ORIENTED_EDGE('',*,*,#43262,.T.);
#56794=ORIENTED_EDGE('',*,*,#43263,.F.);
#56795=ORIENTED_EDGE('',*,*,#43237,.F.);
#56796=ORIENTED_EDGE('',*,*,#43264,.T.);
#56797=ORIENTED_EDGE('',*,*,#43261,.T.);
#56798=ORIENTED_EDGE('',*,*,#43258,.T.);
#56799=ORIENTED_EDGE('',*,*,#43265,.F.);
#56800=ORIENTED_EDGE('',*,*,#43247,.T.);
#56801=ORIENTED_EDGE('',*,*,#43266,.T.);
#56802=ORIENTED_EDGE('',*,*,#43251,.F.);
#56803=ORIENTED_EDGE('',*,*,#43267,.F.);
#56804=ORIENTED_EDGE('',*,*,#43238,.T.);
#56805=ORIENTED_EDGE('',*,*,#43265,.T.);
#56806=ORIENTED_EDGE('',*,*,#43257,.F.);
#56807=ORIENTED_EDGE('',*,*,#43268,.F.);
#56808=ORIENTED_EDGE('',*,*,#43236,.T.);
#56809=ORIENTED_EDGE('',*,*,#43269,.T.);
#56810=ORIENTED_EDGE('',*,*,#43262,.F.);
#56811=ORIENTED_EDGE('',*,*,#43264,.F.);
#56812=ORIENTED_EDGE('',*,*,#43256,.T.);
#56813=ORIENTED_EDGE('',*,*,#43270,.F.);
#56814=ORIENTED_EDGE('',*,*,#43239,.F.);
#56815=ORIENTED_EDGE('',*,*,#43268,.T.);
#56816=ORIENTED_EDGE('',*,*,#43263,.T.);
#56817=ORIENTED_EDGE('',*,*,#43269,.F.);
#56818=ORIENTED_EDGE('',*,*,#43235,.F.);
#56819=ORIENTED_EDGE('',*,*,#43271,.T.);
#56820=ORIENTED_EDGE('',*,*,#43249,.F.);
#56821=ORIENTED_EDGE('',*,*,#43271,.F.);
#56822=ORIENTED_EDGE('',*,*,#43234,.T.);
#56823=ORIENTED_EDGE('',*,*,#43272,.T.);
#56824=ORIENTED_EDGE('',*,*,#43242,.T.);
#56825=ORIENTED_EDGE('',*,*,#43273,.T.);
#56826=ORIENTED_EDGE('',*,*,#43253,.F.);
#56827=ORIENTED_EDGE('',*,*,#43274,.F.);
#56828=ORIENTED_EDGE('',*,*,#43250,.F.);
#56829=ORIENTED_EDGE('',*,*,#43272,.F.);
#56830=ORIENTED_EDGE('',*,*,#43248,.T.);
#56831=ORIENTED_EDGE('',*,*,#43267,.T.);
#56832=ORIENTED_EDGE('',*,*,#43241,.T.);
#56833=ORIENTED_EDGE('',*,*,#43275,.T.);
#56834=ORIENTED_EDGE('',*,*,#43254,.F.);
#56835=ORIENTED_EDGE('',*,*,#43273,.F.);
#56836=ORIENTED_EDGE('',*,*,#43252,.F.);
#56837=ORIENTED_EDGE('',*,*,#43266,.F.);
#56838=ORIENTED_EDGE('',*,*,#43246,.T.);
#56839=ORIENTED_EDGE('',*,*,#43243,.T.);
#56840=ORIENTED_EDGE('',*,*,#43274,.T.);
#56841=ORIENTED_EDGE('',*,*,#43240,.T.);
#56842=ORIENTED_EDGE('',*,*,#43270,.T.);
#56843=ORIENTED_EDGE('',*,*,#43255,.F.);
#56844=ORIENTED_EDGE('',*,*,#43275,.F.);
#56845=ORIENTED_EDGE('',*,*,#43245,.F.);
#56846=ORIENTED_EDGE('',*,*,#43229,.T.);
#56847=ORIENTED_EDGE('',*,*,#43227,.F.);
#56848=ORIENTED_EDGE('',*,*,#43276,.T.);
#56849=ORIENTED_EDGE('',*,*,#43277,.T.);
#56850=ORIENTED_EDGE('',*,*,#43212,.T.);
#56851=ORIENTED_EDGE('',*,*,#43221,.T.);
#56852=ORIENTED_EDGE('',*,*,#43217,.T.);
#56853=ORIENTED_EDGE('',*,*,#43230,.F.);
#56854=ORIENTED_EDGE('',*,*,#43278,.T.);
#56855=ORIENTED_EDGE('',*,*,#43184,.T.);
#56856=ORIENTED_EDGE('',*,*,#43276,.F.);
#56857=ORIENTED_EDGE('',*,*,#43233,.F.);
#56858=ORIENTED_EDGE('',*,*,#43232,.F.);
#56859=ORIENTED_EDGE('',*,*,#43200,.F.);
#56860=ORIENTED_EDGE('',*,*,#43199,.F.);
#56861=ORIENTED_EDGE('',*,*,#43279,.T.);
#56862=ORIENTED_EDGE('',*,*,#43190,.F.);
#56863=ORIENTED_EDGE('',*,*,#43226,.F.);
#56864=ORIENTED_EDGE('',*,*,#43188,.F.);
#56865=ORIENTED_EDGE('',*,*,#43185,.F.);
#56866=ORIENTED_EDGE('',*,*,#43280,.F.);
#56867=ORIENTED_EDGE('',*,*,#43209,.F.);
#56868=ORIENTED_EDGE('',*,*,#43206,.F.);
#56869=ORIENTED_EDGE('',*,*,#43203,.F.);
#56870=ORIENTED_EDGE('',*,*,#43281,.F.);
#56871=ORIENTED_EDGE('',*,*,#43279,.F.);
#56872=ORIENTED_EDGE('',*,*,#43198,.F.);
#56873=ORIENTED_EDGE('',*,*,#43282,.F.);
#56874=ORIENTED_EDGE('',*,*,#43191,.F.);
#56875=ORIENTED_EDGE('',*,*,#43281,.T.);
#56876=ORIENTED_EDGE('',*,*,#43197,.F.);
#56877=ORIENTED_EDGE('',*,*,#43196,.F.);
#56878=ORIENTED_EDGE('',*,*,#43283,.F.);
#56879=ORIENTED_EDGE('',*,*,#43282,.T.);
#56880=ORIENTED_EDGE('',*,*,#43213,.F.);
#56881=ORIENTED_EDGE('',*,*,#43277,.F.);
#56882=ORIENTED_EDGE('',*,*,#43183,.T.);
#56883=ORIENTED_EDGE('',*,*,#43182,.T.);
#56884=ORIENTED_EDGE('',*,*,#43187,.T.);
#56885=ORIENTED_EDGE('',*,*,#43225,.T.);
#56886=ORIENTED_EDGE('',*,*,#43192,.T.);
#56887=ORIENTED_EDGE('',*,*,#43283,.T.);
#56888=ORIENTED_EDGE('',*,*,#43195,.F.);
#56889=ORIENTED_EDGE('',*,*,#43194,.F.);
#56890=ORIENTED_EDGE('',*,*,#43205,.F.);
#56891=ORIENTED_EDGE('',*,*,#43208,.F.);
#56892=ORIENTED_EDGE('',*,*,#43210,.F.);
#56893=ORIENTED_EDGE('',*,*,#43280,.T.);
#56894=ORIENTED_EDGE('',*,*,#43278,.F.);
#56895=ORIENTED_EDGE('',*,*,#43231,.T.);
#56896=ORIENTED_EDGE('',*,*,#43223,.F.);
#56897=ORIENTED_EDGE('',*,*,#43222,.F.);
#56898=ORIENTED_EDGE('',*,*,#43214,.F.);
#56899=ORIENTED_EDGE('',*,*,#43202,.T.);
#56900=ORIENTED_EDGE('',*,*,#43218,.F.);
#56901=ORIENTED_EDGE('',*,*,#43260,.T.);
#56902=ORIENTED_EDGE('',*,*,#43220,.F.);
#76184=ADVANCED_FACE('',(#20754),#2237,.F.);
#76185=ADVANCED_FACE('',(#20755),#2238,.F.);
#76186=ADVANCED_FACE('',(#20756),#2239,.F.);
#76187=ADVANCED_FACE('',(#20757),#2240,.F.);
#76188=ADVANCED_FACE('',(#20758),#2241,.F.);
#76189=ADVANCED_FACE('',(#20759),#2242,.F.);
#76190=ADVANCED_FACE('',(#20760),#2243,.F.);
#76191=ADVANCED_FACE('',(#20761),#2244,.F.);
#76192=ADVANCED_FACE('',(#20762),#2245,.F.);
#76193=ADVANCED_FACE('',(#20763),#2246,.F.);
#76194=ADVANCED_FACE('',(#20764),#2247,.F.);
#76195=ADVANCED_FACE('',(#20765),#1944,.F.);
#76196=ADVANCED_FACE('',(#20766),#1945,.T.);
#76197=ADVANCED_FACE('',(#20767),#1946,.T.);
#76198=ADVANCED_FACE('',(#20768),#2248,.T.);
#76199=ADVANCED_FACE('',(#20769),#16994,.T.);
#76200=ADVANCED_FACE('',(#20770),#16995,.T.);
#76201=ADVANCED_FACE('',(#20771),#16996,.T.);
#76202=ADVANCED_FACE('',(#20772),#2249,.T.);
#76203=ADVANCED_FACE('',(#20773),#2250,.T.);
#76204=ADVANCED_FACE('',(#20774),#16997,.T.);
#76205=ADVANCED_FACE('',(#20775),#16998,.T.);
#76206=ADVANCED_FACE('',(#20776),#2251,.T.);
#76207=ADVANCED_FACE('',(#20777),#2252,.T.);
#76208=ADVANCED_FACE('',(#20778),#2253,.T.);
#76209=ADVANCED_FACE('',(#20779),#16999,.T.);
#76210=ADVANCED_FACE('',(#20780,#302),#17000,.T.);
#76211=ADVANCED_FACE('',(#20781),#191,.F.);
#76212=ADVANCED_FACE('',(#20782),#192,.F.);
#76213=ADVANCED_FACE('',(#20783),#193,.F.);
#76214=ADVANCED_FACE('',(#20784),#194,.F.);
#76215=ADVANCED_FACE('',(#20785),#195,.F.);
#76216=ADVANCED_FACE('',(#20786),#196,.F.);
#76217=ADVANCED_FACE('',(#20787),#197,.F.);
#76218=ADVANCED_FACE('',(#20788),#198,.F.);
#76219=ADVANCED_FACE('',(#20789,#303),#17001,.F.);
#76220=ADVANCED_FACE('',(#20790,#304),#17002,.F.);
#79329=CLOSED_SHELL('',(#76184,#76185,#76186,#76187,#76188,#76189,#76190,
#76191,#76192,#76193,#76194,#76195,#76196,#76197,#76198,#76199,#76200,#76201,
#76202,#76203,#76204,#76205,#76206,#76207,#76208,#76209,#76210,#76211,#76212,
#76213,#76214,#76215,#76216,#76217,#76218,#76219,#76220));
#80796=AXIS2_PLACEMENT_3D('',#177995,#89250,#89251);
#80797=AXIS2_PLACEMENT_3D('',#177996,#89252,#89253);
#80798=AXIS2_PLACEMENT_3D('',#178152,#89256,#89257);
#80799=AXIS2_PLACEMENT_3D('',#178318,#89259,#89260);
#80800=AXIS2_PLACEMENT_3D('',#178348,#89262,#89263);
#80801=AXIS2_PLACEMENT_3D('',#178488,#89267,#89268);
#80802=AXIS2_PLACEMENT_3D('',#178567,#89269,#89270);
#80803=AXIS2_PLACEMENT_3D('',#178733,#89272,#89273);
#80804=AXIS2_PLACEMENT_3D('',#178902,#89275,#89276);
#80805=AXIS2_PLACEMENT_3D('',#179061,#89278,#89279);
#80806=AXIS2_PLACEMENT_3D('',#179066,#89281,#89282);
#80807=AXIS2_PLACEMENT_3D('',#179075,#89283,#89284);
#80808=AXIS2_PLACEMENT_3D('',#179077,#89285,#89286);
#80809=AXIS2_PLACEMENT_3D('',#179080,#89288,#89289);
#80810=AXIS2_PLACEMENT_3D('',#179081,#89290,#89291);
#80811=AXIS2_PLACEMENT_3D('',#179210,#89292,#89293);
#80812=AXIS2_PLACEMENT_3D('',#179211,#89294,#89295);
#80813=AXIS2_PLACEMENT_3D('',#179374,#89296,#89297);
#80814=AXIS2_PLACEMENT_3D('',#179395,#89299,#89300);
#80815=AXIS2_PLACEMENT_3D('',#179501,#89301,#89302);
#80816=AXIS2_PLACEMENT_3D('',#179508,#89303,#89304);
#80817=AXIS2_PLACEMENT_3D('',#179514,#89305,#89306);
#80818=AXIS2_PLACEMENT_3D('',#179520,#89307,#89308);
#80819=AXIS2_PLACEMENT_3D('',#179526,#89309,#89310);
#80820=AXIS2_PLACEMENT_3D('',#179532,#89311,#89312);
#80821=AXIS2_PLACEMENT_3D('',#179535,#89314,#89315);
#80822=AXIS2_PLACEMENT_3D('',#179537,#89316,#89317);
#80823=AXIS2_PLACEMENT_3D('',#179542,#89318,#89319);
#80824=AXIS2_PLACEMENT_3D('',#179543,#89320,#89321);
#80825=AXIS2_PLACEMENT_3D('',#179550,#89322,#89323);
#80826=AXIS2_PLACEMENT_3D('',#179556,#89324,#89325);
#80827=AXIS2_PLACEMENT_3D('',#179562,#89326,#89327);
#80828=AXIS2_PLACEMENT_3D('',#179568,#89328,#89329);
#80829=AXIS2_PLACEMENT_3D('',#179574,#89330,#89331);
#80830=AXIS2_PLACEMENT_3D('',#179577,#89333,#89334);
#80831=AXIS2_PLACEMENT_3D('',#179579,#89335,#89336);
#80832=AXIS2_PLACEMENT_3D('',#179584,#89337,#89338);
#80833=AXIS2_PLACEMENT_3D('',#179585,#89339,#89340);
#80834=AXIS2_PLACEMENT_3D('',#179588,#89343,#89344);
#80835=AXIS2_PLACEMENT_3D('',#179591,#89347,#89348);
#80836=AXIS2_PLACEMENT_3D('',#179593,#89350,#89351);
#80837=AXIS2_PLACEMENT_3D('',#179595,#89353,#89354);
#80838=AXIS2_PLACEMENT_3D('',#179597,#89356,#89357);
#80839=AXIS2_PLACEMENT_3D('',#179599,#89359,#89360);
#80840=AXIS2_PLACEMENT_3D('',#179601,#89362,#89363);
#80841=AXIS2_PLACEMENT_3D('',#179604,#89366,#89367);
#80842=AXIS2_PLACEMENT_3D('',#179605,#89368,#89369);
#80843=AXIS2_PLACEMENT_3D('',#179607,#89371,#89372);
#80844=AXIS2_PLACEMENT_3D('',#179608,#89373,#89374);
#80845=AXIS2_PLACEMENT_3D('',#179609,#89375,#89376);
#80846=AXIS2_PLACEMENT_3D('',#181108,#89379,#89380);
#80847=AXIS2_PLACEMENT_3D('',#181109,#89381,#89382);
#89250=DIRECTION('axis',(0.,0.,1.));
#89251=DIRECTION('refdir',(1.,0.,0.));
#89252=DIRECTION('center_axis',(-1.,0.,0.));
#89253=DIRECTION('ref_axis',(0.,0.,1.));
#89254=DIRECTION('',(-1.,0.,0.));
#89255=DIRECTION('',(-0.999999999965599,-7.79366990386846E-6,-2.8389956576918E-6));
#89256=DIRECTION('center_axis',(-1.,0.,0.));
#89257=DIRECTION('ref_axis',(0.,0.,1.));
#89258=DIRECTION('',(-1.,0.,0.));
#89259=DIRECTION('center_axis',(-1.,0.,0.));
#89260=DIRECTION('ref_axis',(0.,0.,1.));
#89261=DIRECTION('',(-1.,0.,0.));
#89262=DIRECTION('center_axis',(1.,0.,0.));
#89263=DIRECTION('ref_axis',(0.,0.,-1.));
#89264=DIRECTION('',(1.,0.,0.));
#89265=DIRECTION('',(0.999999999992329,-8.06779552607498E-7,3.8330006150557E-6));
#89266=DIRECTION('',(1.,0.,0.));
#89267=DIRECTION('center_axis',(-1.,0.,0.));
#89268=DIRECTION('ref_axis',(0.,1.,0.));
#89269=DIRECTION('center_axis',(1.,0.,0.));
#89270=DIRECTION('ref_axis',(0.,0.,-1.));
#89271=DIRECTION('',(1.,0.,0.));
#89272=DIRECTION('center_axis',(1.,0.,0.));
#89273=DIRECTION('ref_axis',(0.,0.,-1.));
#89274=DIRECTION('',(1.,0.,0.));
#89275=DIRECTION('center_axis',(1.,0.,0.));
#89276=DIRECTION('ref_axis',(0.,0.,-1.));
#89277=DIRECTION('',(1.,0.,0.));
#89278=DIRECTION('center_axis',(1.,0.,0.));
#89279=DIRECTION('ref_axis',(0.,0.,-1.));
#89280=DIRECTION('',(1.,0.,0.));
#89281=DIRECTION('center_axis',(-1.,0.,0.));
#89282=DIRECTION('ref_axis',(0.,-0.957773424896036,-0.287524027801011));
#89283=DIRECTION('center_axis',(1.,0.,0.));
#89284=DIRECTION('ref_axis',(0.,0.,-1.));
#89285=DIRECTION('center_axis',(-1.,0.,0.));
#89286=DIRECTION('ref_axis',(0.,1.,0.));
#89287=DIRECTION('',(1.,0.,0.));
#89288=DIRECTION('center_axis',(1.,0.,0.));
#89289=DIRECTION('ref_axis',(0.,-1.,0.));
#89290=DIRECTION('center_axis',(1.,0.,0.));
#89291=DIRECTION('ref_axis',(0.,0.,-1.));
#89292=DIRECTION('center_axis',(-1.,0.,0.));
#89293=DIRECTION('ref_axis',(0.,-0.957773424896036,-0.287524027801011));
#89294=DIRECTION('center_axis',(-1.,0.,0.));
#89295=DIRECTION('ref_axis',(0.,0.,1.));
#89296=DIRECTION('center_axis',(-1.,0.,8.90699599727784E-17));
#89297=DIRECTION('ref_axis',(8.90699599727784E-17,0.,1.));
#89298=DIRECTION('',(-0.707106708341652,-8.65956145444752E-17,-0.707106854031435));
#89299=DIRECTION('center_axis',(1.,0.,0.));
#89300=DIRECTION('ref_axis',(0.,1.,0.));
#89301=DIRECTION('center_axis',(1.,0.,-6.83634867380023E-18));
#89302=DIRECTION('ref_axis',(-6.83634867380023E-18,0.,-1.));
#89303=DIRECTION('center_axis',(-1.,0.,0.));
#89304=DIRECTION('ref_axis',(0.,0.906250000000018,-0.422742164327108));
#89305=DIRECTION('center_axis',(-1.,0.,0.));
#89306=DIRECTION('ref_axis',(0.,0.087019546441882,-0.99620660434322));
#89307=DIRECTION('center_axis',(-1.,0.,0.));
#89308=DIRECTION('ref_axis',(0.,-0.819230453558104,-0.573464440016103));
#89309=DIRECTION('center_axis',(1.,0.,0.));
#89310=DIRECTION('ref_axis',(0.,-0.819230453558104,0.573464440016103));
#89311=DIRECTION('center_axis',(1.,0.,0.));
#89312=DIRECTION('ref_axis',(0.,0.087019546441882,0.99620660434322));
#89313=DIRECTION('',(-0.707106781821139,8.65956055458343E-17,-0.707106780551956));
#89314=DIRECTION('center_axis',(1.,0.,0.));
#89315=DIRECTION('ref_axis',(0.,-1.,0.));
#89316=DIRECTION('center_axis',(1.,0.,0.));
#89317=DIRECTION('ref_axis',(0.,0.087019546441882,0.99620660434322));
#89318=DIRECTION('center_axis',(1.,0.,0.));
#89319=DIRECTION('ref_axis',(0.,0.906250000000018,0.422742164327108));
#89320=DIRECTION('center_axis',(-1.,0.,-1.02545230107003E-16));
#89321=DIRECTION('ref_axis',(-1.02545230107003E-16,0.,1.));
#89322=DIRECTION('center_axis',(1.,0.,0.));
#89323=DIRECTION('ref_axis',(0.,0.906250000000018,0.422742164327108));
#89324=DIRECTION('center_axis',(1.,0.,0.));
#89325=DIRECTION('ref_axis',(0.,0.087019546441882,0.99620660434322));
#89326=DIRECTION('center_axis',(1.,0.,0.));
#89327=DIRECTION('ref_axis',(0.,-0.819230453558104,0.573464440016103));
#89328=DIRECTION('center_axis',(-1.,0.,0.));
#89329=DIRECTION('ref_axis',(0.,-0.819230453558104,-0.573464440016103));
#89330=DIRECTION('center_axis',(-1.,0.,0.));
#89331=DIRECTION('ref_axis',(0.,0.087019546441882,-0.99620660434322));
#89332=DIRECTION('',(0.707106781821139,8.65956055458343E-17,0.707106780551956));
#89333=DIRECTION('center_axis',(1.,0.,0.));
#89334=DIRECTION('ref_axis',(0.,1.,0.));
#89335=DIRECTION('center_axis',(-1.,0.,0.));
#89336=DIRECTION('ref_axis',(0.,0.087019546441882,-0.99620660434322));
#89337=DIRECTION('center_axis',(-1.,0.,0.));
#89338=DIRECTION('ref_axis',(0.,0.906250000000018,-0.422742164327108));
#89339=DIRECTION('center_axis',(1.,0.,0.));
#89340=DIRECTION('ref_axis',(0.,0.,-1.));
#89341=DIRECTION('',(1.,0.,0.));
#89342=DIRECTION('',(1.,0.,0.));
#89343=DIRECTION('center_axis',(0.,0.500000000000017,0.866025403784429));
#89344=DIRECTION('ref_axis',(1.,0.,0.));
#89345=DIRECTION('',(1.,0.,0.));
#89346=DIRECTION('',(1.,0.,0.));
#89347=DIRECTION('center_axis',(0.,-0.500000000000017,-0.866025403784429));
#89348=DIRECTION('ref_axis',(0.,-0.866025403784429,0.500000000000017));
#89349=DIRECTION('',(1.,0.,0.));
#89350=DIRECTION('center_axis',(0.,0.500000000000017,-0.866025403784429));
#89351=DIRECTION('ref_axis',(-1.,0.,0.));
#89352=DIRECTION('',(1.,0.,0.));
#89353=DIRECTION('center_axis',(1.,0.,0.));
#89354=DIRECTION('ref_axis',(0.,0.,-1.));
#89355=DIRECTION('',(1.,0.,0.));
#89356=DIRECTION('center_axis',(1.,0.,0.));
#89357=DIRECTION('ref_axis',(0.,0.,-1.));
#89358=DIRECTION('',(1.,0.,0.));
#89359=DIRECTION('center_axis',(0.,1.,0.));
#89360=DIRECTION('ref_axis',(1.,0.,0.));
#89361=DIRECTION('',(1.,0.,0.));
#89362=DIRECTION('center_axis',(0.,-0.500000000000017,0.866025403784429));
#89363=DIRECTION('ref_axis',(-1.,0.,0.));
#89364=DIRECTION('',(1.,0.,0.));
#89365=DIRECTION('',(1.,0.,0.));
#89366=DIRECTION('center_axis',(1.,0.,0.));
#89367=DIRECTION('ref_axis',(0.,0.,-1.));
#89368=DIRECTION('center_axis',(1.,0.,0.));
#89369=DIRECTION('ref_axis',(0.,0.,-1.));
#89370=DIRECTION('',(1.,0.,0.));
#89371=DIRECTION('center_axis',(1.,0.,0.));
#89372=DIRECTION('ref_axis',(0.,-5.35449122399261E-13,1.));
#89373=DIRECTION('center_axis',(0.,-1.,0.));
#89374=DIRECTION('ref_axis',(0.,0.,-1.));
#89375=DIRECTION('center_axis',(-1.,0.,0.));
#89376=DIRECTION('ref_axis',(0.,0.,1.));
#89377=DIRECTION('',(-0.461790830635516,-0.303368053954436,0.833496882166249));
#89378=DIRECTION('',(-0.461753481727666,0.303366050430997,-0.833518303073349));
#89379=DIRECTION('center_axis',(1.,0.,0.));
#89380=DIRECTION('ref_axis',(0.,1.,0.));
#89381=DIRECTION('center_axis',(-1.,0.,0.));
#89382=DIRECTION('ref_axis',(0.,0.,1.));
#177995=CARTESIAN_POINT('',(0.,0.,0.));
#177996=CARTESIAN_POINT('Origin',(-23.90845228375,-75.0031087425464,72.9873550812444));
#177997=CARTESIAN_POINT('',(-23.2177969711981,-75.0031087425464,59.9387052680259));
#177998=CARTESIAN_POINT('',(-23.5174110875174,-75.0031087425464,59.9387052680259));
#177999=CARTESIAN_POINT('',(-23.90845228375,-75.0031087425464,59.9387052680259));
#178000=CARTESIAN_POINT('',(-24.4189072313413,-75.0031417059253,86.0360048944213));
#178001=CARTESIAN_POINT('Ctrl Pts',(-23.5174110875174,-75.0031087425464,
59.9387052680259));
#178002=CARTESIAN_POINT('Ctrl Pts',(-23.5258740395449,-75.3885856088758,
59.9387052680259));
#178003=CARTESIAN_POINT('Ctrl Pts',(-23.5343495220848,-75.7740190949249,
59.9557866063909));
#178004=CARTESIAN_POINT('Ctrl Pts',(-23.5617944162149,-77.0283277708885,
60.067265150459));
#178005=CARTESIAN_POINT('Ctrl Pts',(-23.5806373594291,-77.8884227880291,
60.2317600988326));
#178006=CARTESIAN_POINT('Ctrl Pts',(-23.6089443886813,-79.1242668073003,
60.5996061157332));
#178007=CARTESIAN_POINT('Ctrl Pts',(-23.6181074284407,-79.5170208469362,
60.7372585206103));
#178008=CARTESIAN_POINT('Ctrl Pts',(-23.6431780322771,-80.5789266596909,
61.1674516227681));
#178009=CARTESIAN_POINT('Ctrl Pts',(-23.6589117584693,-81.2311459690073,
61.497732867221));
#178010=CARTESIAN_POINT('Ctrl Pts',(-23.68934766305,-82.414672015085,62.2275925132549));
#178011=CARTESIAN_POINT('Ctrl Pts',(-23.7039535895129,-82.9498688086055,
62.616590314994));
#178012=CARTESIAN_POINT('Ctrl Pts',(-23.7347491794576,-84.0220013905403,
63.5277639727065));
#178013=CARTESIAN_POINT('Ctrl Pts',(-23.7508786121394,-84.5481913996176,
64.0589906959572));
#178014=CARTESIAN_POINT('Ctrl Pts',(-23.7819901432446,-85.4556145331789,
65.1475589814397));
#178015=CARTESIAN_POINT('Ctrl Pts',(-23.7968526295174,-85.8447759766575,
65.6951994335084));
#178016=CARTESIAN_POINT('Ctrl Pts',(-23.8226701199644,-86.452147742019,
66.706757312822));
#178017=CARTESIAN_POINT('Ctrl Pts',(-23.8337287308387,-86.6884310827492,
67.1581488692751));
#178018=CARTESIAN_POINT('Ctrl Pts',(-23.8637678447263,-87.2523286094977,
68.4083152461614));
#178019=CARTESIAN_POINT('Ctrl Pts',(-23.882921492897,-87.5281114458154,
69.22766109732));
#178020=CARTESIAN_POINT('Ctrl Pts',(-23.9138265338306,-87.8435897107306,
70.6021111891274));
#178021=CARTESIAN_POINT('Ctrl Pts',(-23.9257488716751,-87.9323958052821,
71.1432084592251));
#178022=CARTESIAN_POINT('Ctrl Pts',(-23.9524410857355,-88.0533393736483,
72.352000542165));
#178023=CARTESIAN_POINT('Ctrl Pts',(-23.9672449577233,-88.068755849995,
73.0198351480965));
#178024=CARTESIAN_POINT('Ctrl Pts',(-24.0010417074449,-87.9867815343067,
74.5488835393699));
#178025=CARTESIAN_POINT('Ctrl Pts',(-24.0197803191019,-87.8548981206235,
75.4051312796587));
#178026=CARTESIAN_POINT('Ctrl Pts',(-24.057933133333,-87.4242752312913,
77.0770172011696));
#178027=CARTESIAN_POINT('Ctrl Pts',(-24.0770391433777,-87.1269764979674,
77.8886355774496));
#178028=CARTESIAN_POINT('Ctrl Pts',(-24.1052341797259,-86.5675808489017,
79.0461925561804));
#178029=CARTESIAN_POINT('Ctrl Pts',(-24.1145281505967,-86.3649112316087,
79.4182158163765));
#178030=CARTESIAN_POINT('Ctrl Pts',(-24.1388756575297,-85.7912380572986,
80.3592018984337));
#178031=CARTESIAN_POINT('Ctrl Pts',(-24.1540139134244,-85.3932895243157,
80.9102335930352));
#178032=CARTESIAN_POINT('Ctrl Pts',(-24.1885571156498,-84.3793035702454,
82.1057102021331));
#178033=CARTESIAN_POINT('Ctrl Pts',(-24.2079565921027,-83.7365453105005,
82.723089235518));
#178034=CARTESIAN_POINT('Ctrl Pts',(-24.2355717066776,-82.7562314143682,
83.4888987406805));
#178035=CARTESIAN_POINT('Ctrl Pts',(-24.2434729123377,-82.4676211814838,
83.6959677129961));
#178036=CARTESIAN_POINT('Ctrl Pts',(-24.2704762780277,-81.4487495403035,
84.365751152243));
#178037=CARTESIAN_POINT('Ctrl Pts',(-24.2892701843075,-80.6811917885786,
84.7675739845685));
#178038=CARTESIAN_POINT('Ctrl Pts',(-24.326542154466,-79.1204700528668,
85.3963986786834));
#178039=CARTESIAN_POINT('Ctrl Pts',(-24.3447363405948,-78.3342799627899,
85.6301527642972));
#178040=CARTESIAN_POINT('Ctrl Pts',(-24.3813496645858,-76.6986863541472,
85.9531842222863));
#178041=CARTESIAN_POINT('Ctrl Pts',(-24.4000561482487,-75.8519283269992,
86.0360027502243));
#178042=CARTESIAN_POINT('Ctrl Pts',(-24.4189072313414,-75.0031417059253,
86.0360048944213));
#178043=CARTESIAN_POINT('',(-25.2173493892328,-70.5370130173974,60.7268819234023));
#178044=CARTESIAN_POINT('Ctrl Pts',(-25.2179534601443,-70.5369625382682,
60.7268167557867));
#178045=CARTESIAN_POINT('Ctrl Pts',(-25.1949255782263,-69.5510845400866,
61.0859425268238));
#178046=CARTESIAN_POINT('Ctrl Pts',(-25.1723485468244,-68.6121132844695,
61.5626729666513));
#178047=CARTESIAN_POINT('Ctrl Pts',(-25.1418319224832,-67.4503279249558,
62.3410093155562));
#178048=CARTESIAN_POINT('Ctrl Pts',(-25.1341597941179,-67.168164933375,
62.546912976461));
#178049=CARTESIAN_POINT('Ctrl Pts',(-25.1058958914003,-66.1590701068227,
63.3472530553906));
#178050=CARTESIAN_POINT('Ctrl Pts',(-25.0856284897384,-65.4886400931649,
64.0082978440766));
#178051=CARTESIAN_POINT('Ctrl Pts',(-25.0463381621821,-64.3476753322238,
65.4059328423162));
#178052=CARTESIAN_POINT('Ctrl Pts',(-25.0272324006768,-63.8684396267926,
66.1291213644448));
#178053=CARTESIAN_POINT('Ctrl Pts',(-24.9900396375432,-63.0713109933876,
67.638717086007));
#178054=CARTESIAN_POINT('Ctrl Pts',(-24.9718326777438,-62.7512240802528,
68.4193091338589));
#178055=CARTESIAN_POINT('Ctrl Pts',(-24.9272869194739,-62.167302597689,
70.3586157342146));
#178056=CARTESIAN_POINT('Ctrl Pts',(-24.9018234838554,-61.9818391597063,
71.5331436490922));
#178057=CARTESIAN_POINT('Ctrl Pts',(-24.8571030316205,-61.939606164877,
73.5672948670295));
#178058=CARTESIAN_POINT('Ctrl Pts',(-24.8383743123942,-62.0052128063284,
74.4177895566878));
#178059=CARTESIAN_POINT('Ctrl Pts',(-24.8106986129752,-62.2258618857267,
75.6676798065923));
#178060=CARTESIAN_POINT('Ctrl Pts',(-24.8016093736651,-62.3183287152197,
76.0758065751899));
#178061=CARTESIAN_POINT('Ctrl Pts',(-24.7773198416253,-62.6143520358101,
77.1418062935212));
#178062=CARTESIAN_POINT('Ctrl Pts',(-24.7620753388425,-62.8506276162574,
77.7892260852831));
#178063=CARTESIAN_POINT('Ctrl Pts',(-24.730838002126,-63.4428299151513,
79.083938962895));
#178064=CARTESIAN_POINT('Ctrl Pts',(-24.7149083735733,-63.8048278788549,
79.7258182827486));
#178065=CARTESIAN_POINT('Ctrl Pts',(-24.687301631946,-64.509686240891,80.7605121738516));
#178066=CARTESIAN_POINT('Ctrl Pts',(-24.6758558722316,-64.8254709287872,
81.169627195189));
#178067=CARTESIAN_POINT('Ctrl Pts',(-24.6475001697529,-65.6709139270774,
82.1400231901055));
#178068=CARTESIAN_POINT('Ctrl Pts',(-24.6307810261119,-66.2276452856273,
82.6751014390459));
#178069=CARTESIAN_POINT('Ctrl Pts',(-24.5995857708681,-67.3310996828718,
83.5620240742223));
#178070=CARTESIAN_POINT('Ctrl Pts',(-24.5852411678063,-67.8631451133042,
83.9282997510201));
#178071=CARTESIAN_POINT('Ctrl Pts',(-24.5583913263179,-68.9148227684136,
84.5428023817671));
#178072=CARTESIAN_POINT('Ctrl Pts',(-24.5458806664972,-69.42805990607,84.7989772586328));
#178073=CARTESIAN_POINT('Ctrl Pts',(-24.514390222347,-70.7504543245645,
85.3535788428957));
#178074=CARTESIAN_POINT('Ctrl Pts',(-24.4951894160082,-71.5754500366103,
85.607169318098));
#178075=CARTESIAN_POINT('Ctrl Pts',(-24.4570936740862,-73.2699077150253,
85.9494606259919));
#178076=CARTESIAN_POINT('Ctrl Pts',(-24.4381782821793,-74.1354456671949,
86.036007086387));
#178077=CARTESIAN_POINT('Ctrl Pts',(-24.4189072313414,-75.0031417059253,
86.0360048944213));
#178078=CARTESIAN_POINT('',(-24.9173192207092,-70.5369340980989,60.7267130748814));
#178079=CARTESIAN_POINT('',(-24.9176605481234,-70.5369675179446,60.7268149418411));
#178080=CARTESIAN_POINT('Ctrl Pts',(-24.9171176851385,-70.5369733775824,
60.7268128073552));
#178081=CARTESIAN_POINT('Ctrl Pts',(-24.907354037465,-70.1192429353976,
60.8789790540991));
#178082=CARTESIAN_POINT('Ctrl Pts',(-24.8975797564189,-69.7095626266936,
61.0523944958426));
#178083=CARTESIAN_POINT('Ctrl Pts',(-24.8780421092287,-68.915232029882,
61.4375907871025));
#178084=CARTESIAN_POINT('Ctrl Pts',(-24.8682932702408,-68.5308118305049,
61.64854254573));
#178085=CARTESIAN_POINT('Ctrl Pts',(-24.839312347075,-67.4195428302757,
62.3333119862464));
#178086=CARTESIAN_POINT('Ctrl Pts',(-24.8204486087593,-66.7285259145455,
62.8606386207108));
#178087=CARTESIAN_POINT('Ctrl Pts',(-24.7870712095047,-65.6249880349399,
63.8916559887359));
#178088=CARTESIAN_POINT('Ctrl Pts',(-24.7727296370073,-65.1881453816324,
64.3648623656643));
#178089=CARTESIAN_POINT('Ctrl Pts',(-24.742250830614,-64.3297071453802,
65.4449268297063));
#178090=CARTESIAN_POINT('Ctrl Pts',(-24.7262134284685,-63.9210741808339,
66.0592788242168));
#178091=CARTESIAN_POINT('Ctrl Pts',(-24.6980302381648,-63.3069294808542,
67.1772593829506));
#178092=CARTESIAN_POINT('Ctrl Pts',(-24.6860398778007,-63.076924372585,
67.6653304883622));
#178093=CARTESIAN_POINT('Ctrl Pts',(-24.6549461700741,-62.5579145370382,
68.9706612988227));
#178094=CARTESIAN_POINT('Ctrl Pts',(-24.6361603086848,-62.318910108264,
69.8049355406911));
#178095=CARTESIAN_POINT('Ctrl Pts',(-24.5983722391606,-62.0133377431336,
71.4882412958202));
#178096=CARTESIAN_POINT('Ctrl Pts',(-24.5796277914179,-61.9435284678936,
72.3324777567359));
#178097=CARTESIAN_POINT('Ctrl Pts',(-24.5427656769566,-61.9680684749626,
74.0162199068147));
#178098=CARTESIAN_POINT('Ctrl Pts',(-24.5243480055858,-62.0611344834041,
74.8517940532979));
#178099=CARTESIAN_POINT('Ctrl Pts',(-24.4878677169977,-62.4004662751921,
76.46542723281));
#178100=CARTESIAN_POINT('Ctrl Pts',(-24.4702471435588,-62.640654323058,
77.2409779439216));
#178101=CARTESIAN_POINT('Ctrl Pts',(-24.433796255826,-63.2784289509455,
78.7776809955811));
#178102=CARTESIAN_POINT('Ctrl Pts',(-24.4148532855467,-63.6822389597166,
79.5321159405294));
#178103=CARTESIAN_POINT('Ctrl Pts',(-24.3870337108765,-64.3884638652798,
80.5880248805467));
#178104=CARTESIAN_POINT('Ctrl Pts',(-24.3779772084299,-64.6365595877853,
80.9230672036952));
#178105=CARTESIAN_POINT('Ctrl Pts',(-24.3526031268852,-65.3720877557516,
81.8228797791645));
#178106=CARTESIAN_POINT('Ctrl Pts',(-24.3361839511979,-65.8925173725387,
82.3585972053378));
#178107=CARTESIAN_POINT('Ctrl Pts',(-24.3007805274961,-67.1080018457081,
83.4123021007472));
#178108=CARTESIAN_POINT('Ctrl Pts',(-24.2821791710908,-67.8146617871703,
83.9115696836482));
#178109=CARTESIAN_POINT('Ctrl Pts',(-24.2540944650781,-68.9301293119283,
84.5442570908524));
#178110=CARTESIAN_POINT('Ctrl Pts',(-24.2448678542072,-69.3045934236883,
84.7334176271645));
#178111=CARTESIAN_POINT('Ctrl Pts',(-24.216668816178,-70.4754509318188,
85.2556863772761));
#178112=CARTESIAN_POINT('Ctrl Pts',(-24.1980647980835,-71.2963084756696,
85.5281394442645));
#178113=CARTESIAN_POINT('Ctrl Pts',(-24.163396596036,-72.8455498637824,
85.8768137532399));
#178114=CARTESIAN_POINT('Ctrl Pts',(-24.1473926977216,-73.5651139084155,
85.9767881417826));
#178115=CARTESIAN_POINT('Ctrl Pts',(-24.1158008336593,-75.010197341672,
86.0559642583735));
#178116=CARTESIAN_POINT('Ctrl Pts',(-24.1002471628222,-75.733187632082,
86.0355574927849));
#178117=CARTESIAN_POINT('Ctrl Pts',(-24.0657733724578,-77.301063771048,
85.8605317011928));
#178118=CARTESIAN_POINT('Ctrl Pts',(-24.0469468205147,-78.1399678374923,
85.6822121490468));
#178119=CARTESIAN_POINT('Ctrl Pts',(-24.010189394764,-79.7547398415525,
85.1690140982003));
#178120=CARTESIAN_POINT('Ctrl Pts',(-23.9919616414302,-80.527762820596,
84.8384734047039));
#178121=CARTESIAN_POINT('Ctrl Pts',(-23.9546341481889,-82.0200678806927,
84.0224231758214));
#178122=CARTESIAN_POINT('Ctrl Pts',(-23.9360244917028,-82.7335970089921,
83.5348665781671));
#178123=CARTESIAN_POINT('Ctrl Pts',(-23.8989792941308,-84.0370277063888,
82.4404483463286));
#178124=CARTESIAN_POINT('Ctrl Pts',(-23.8804521106617,-84.6265974673046,
81.8395370520967));
#178125=CARTESIAN_POINT('Ctrl Pts',(-23.8471181138764,-85.5882146151588,
80.6489263907446));
#178126=CARTESIAN_POINT('Ctrl Pts',(-23.8322209852127,-85.9787829923853,
80.0781038763657));
#178127=CARTESIAN_POINT('Ctrl Pts',(-23.798456560602,-86.7469237694405,
78.7387393171392));
#178128=CARTESIAN_POINT('Ctrl Pts',(-23.7796666603123,-87.0978561620125,
77.9585423880256));
#178129=CARTESIAN_POINT('Ctrl Pts',(-23.742885269507,-87.6378737949811,
76.3540605202281));
#178130=CARTESIAN_POINT('Ctrl Pts',(-23.7245943383307,-87.8282524332701,
75.5344466062342));
#178131=CARTESIAN_POINT('Ctrl Pts',(-23.6888150613604,-88.0419621207994,
73.922431733533));
#178132=CARTESIAN_POINT('Ctrl Pts',(-23.671751351237,-88.074616373477,73.1348591085154));
#178133=CARTESIAN_POINT('Ctrl Pts',(-23.6366919564938,-87.9960084407066,
71.529557093911));
#178134=CARTESIAN_POINT('Ctrl Pts',(-23.6185648586246,-87.878651766991,
70.7155723503837));
#178135=CARTESIAN_POINT('Ctrl Pts',(-23.5861034257923,-87.5307434037802,
69.2780105212558));
#178136=CARTESIAN_POINT('Ctrl Pts',(-23.5718543535404,-87.3276283875879,
68.6506414981074));
#178137=CARTESIAN_POINT('Ctrl Pts',(-23.5481237056837,-86.9171444844969,
67.6485192350802));
#178138=CARTESIAN_POINT('Ctrl Pts',(-23.5387724395496,-86.7371913800963,
67.2638317826352));
#178139=CARTESIAN_POINT('Ctrl Pts',(-23.5103596573091,-86.1358175788794,
66.1263420779984));
#178140=CARTESIAN_POINT('Ctrl Pts',(-23.4916029113219,-85.6582590297536,
65.4058986222406));
#178141=CARTESIAN_POINT('Ctrl Pts',(-23.4537955479461,-84.5678435881823,
64.0695602513784));
#178142=CARTESIAN_POINT('Ctrl Pts',(-23.4346204906349,-83.9576249067465,
63.4569902583999));
#178143=CARTESIAN_POINT('Ctrl Pts',(-23.4005635230591,-82.7595073227506,
62.4716583259945));
#178144=CARTESIAN_POINT('Ctrl Pts',(-23.3855753038685,-82.1937684308081,
62.0769924688238));
#178145=CARTESIAN_POINT('Ctrl Pts',(-23.3517305051871,-80.8700308021691,
61.3014086187056));
#178146=CARTESIAN_POINT('Ctrl Pts',(-23.3329524032564,-80.100710066655,
60.9459022531436));
#178147=CARTESIAN_POINT('Ctrl Pts',(-23.2958780198951,-78.5039024588121,
60.3886648378157));
#178148=CARTESIAN_POINT('Ctrl Pts',(-23.2772858870629,-77.6801776269435,
60.1882985938689));
#178149=CARTESIAN_POINT('Ctrl Pts',(-23.244844685141,-76.2331614615956,
59.98222025733));
#178150=CARTESIAN_POINT('Ctrl Pts',(-23.2313015712184,-75.6183651000271,
59.9387052680259));
#178151=CARTESIAN_POINT('Ctrl Pts',(-23.2177969711981,-75.0031087425464,
59.9387052680259));
#178152=CARTESIAN_POINT('Origin',(-23.90845228375,-75.0031087425464,72.9873550812444));
#178153=CARTESIAN_POINT('',(-21.4178560137238,-75.0031087387644,59.9387052680259));
#178154=CARTESIAN_POINT('',(-21.7173525905574,-75.0031087425464,59.9387052680259));
#178155=CARTESIAN_POINT('',(-23.90845228375,-75.0031087425464,59.9387052680259));
#178156=CARTESIAN_POINT('Ctrl Pts',(-21.7173525905574,-75.0031087425464,
59.9387052680259));
#178157=CARTESIAN_POINT('Ctrl Pts',(-21.7279055222494,-75.4850294936703,
59.9387052680259));
#178158=CARTESIAN_POINT('Ctrl Pts',(-21.7385230017382,-75.9668862553294,
59.9654031749341));
#178159=CARTESIAN_POINT('Ctrl Pts',(-21.7679240675029,-77.3024452901014,
60.1140452558455));
#178160=CARTESIAN_POINT('Ctrl Pts',(-21.7864421216113,-78.1469014580676,
60.2938282072216));
#178161=CARTESIAN_POINT('Ctrl Pts',(-21.8159352477052,-79.4291237185252,
60.702712051699));
#178162=CARTESIAN_POINT('Ctrl Pts',(-21.8266151492676,-79.882222448103,
60.8755298104572));
#178163=CARTESIAN_POINT('Ctrl Pts',(-21.8519577830707,-80.9380865230419,
61.3471373671513));
#178164=CARTESIAN_POINT('Ctrl Pts',(-21.8664533772828,-81.5294397994638,
61.6680956779007));
#178165=CARTESIAN_POINT('Ctrl Pts',(-21.9000034898083,-82.8187825234477,
62.5026496888453));
#178166=CARTESIAN_POINT('Ctrl Pts',(-21.9191269729969,-83.4957006312058,
63.043025618808));
#178167=CARTESIAN_POINT('Ctrl Pts',(-21.9473475391778,-84.4216993305954,
63.9462324866392));
#178168=CARTESIAN_POINT('Ctrl Pts',(-21.9566752112369,-84.7141784534085,
64.2611375895916));
#178169=CARTESIAN_POINT('Ctrl Pts',(-21.9833264542847,-85.4990775401469,
65.1946537624708));
#178170=CARTESIAN_POINT('Ctrl Pts',(-22.0008084882079,-85.951579087771,
65.8443486378435));
#178171=CARTESIAN_POINT('Ctrl Pts',(-22.0325838201198,-86.6674665002242,
67.101668350843));
#178172=CARTESIAN_POINT('Ctrl Pts',(-22.0468106480542,-86.9488626352141,
67.6960871336582));
#178173=CARTESIAN_POINT('Ctrl Pts',(-22.0777047614038,-87.4537260096757,
69.0106622728197));
#178174=CARTESIAN_POINT('Ctrl Pts',(-22.0943914982232,-87.6620372687037,
69.7341288886568));
#178175=CARTESIAN_POINT('Ctrl Pts',(-22.1294675642277,-87.9700062664921,
71.3014524052135));
#178176=CARTESIAN_POINT('Ctrl Pts',(-22.147833465954,-88.0520039394007,
72.145310832488));
#178177=CARTESIAN_POINT('Ctrl Pts',(-22.1756984054644,-88.0516373226961,
73.4062056611231));
#178178=CARTESIAN_POINT('Ctrl Pts',(-22.1849086029447,-88.0317133004347,
73.8210197869936));
#178179=CARTESIAN_POINT('Ctrl Pts',(-22.2165499231349,-87.8947925396264,
75.2474115217725));
#178180=CARTESIAN_POINT('Ctrl Pts',(-22.2386139872856,-87.6793050389978,
76.2457925937928));
#178181=CARTESIAN_POINT('Ctrl Pts',(-22.2704084912974,-87.2151472936438,
77.6033153361541));
#178182=CARTESIAN_POINT('Ctrl Pts',(-22.2796727141446,-87.0614873053053,
77.9910019193931));
#178183=CARTESIAN_POINT('Ctrl Pts',(-22.3051887888618,-86.5841101656086,
79.0450571324956));
#178184=CARTESIAN_POINT('Ctrl Pts',(-22.3213071119102,-86.2218425641866,
79.692231264384));
#178185=CARTESIAN_POINT('Ctrl Pts',(-22.3529083373018,-85.4201163206346,
80.8758455797193));
#178186=CARTESIAN_POINT('Ctrl Pts',(-22.3682834493315,-84.9889684320517,
81.4149845564498));
#178187=CARTESIAN_POINT('Ctrl Pts',(-22.3950863482788,-84.1558584102784,
82.3025736978643));
#178188=CARTESIAN_POINT('Ctrl Pts',(-22.4066316775564,-83.7714168305926,
82.6653145011311));
#178189=CARTESIAN_POINT('Ctrl Pts',(-22.4338912775281,-82.8225075887755,
83.4575825212767));
#178190=CARTESIAN_POINT('Ctrl Pts',(-22.4496709708313,-82.2429225410224,
83.8664060700109));
#178191=CARTESIAN_POINT('Ctrl Pts',(-22.4826037731214,-80.9612295771777,
84.6224938354518));
#178192=CARTESIAN_POINT('Ctrl Pts',(-22.4995831787795,-80.2552331908446,
84.9577706620152));
#178193=CARTESIAN_POINT('Ctrl Pts',(-22.5325450616795,-78.8574394922688,
85.4739714605351));
#178194=CARTESIAN_POINT('Ctrl Pts',(-22.5483954088286,-78.1723752269056,
85.665178554888));
#178195=CARTESIAN_POINT('Ctrl Pts',(-22.5760360101624,-76.9397628278786,
85.903003010317));
#178196=CARTESIAN_POINT('Ctrl Pts',(-22.587959276298,-76.3984101366401,
85.9726438876509));
#178197=CARTESIAN_POINT('Ctrl Pts',(-22.6190042307515,-74.9942563843571,
86.0644345013557));
#178198=CARTESIAN_POINT('Ctrl Pts',(-22.6382386174052,-74.1307621203506,
86.0353089734078));
#178199=CARTESIAN_POINT('Ctrl Pts',(-22.6727313652882,-72.5749278003073,
85.8276092401245));
#178200=CARTESIAN_POINT('Ctrl Pts',(-22.688208923268,-71.8821713248205,
85.6770335192465));
#178201=CARTESIAN_POINT('Ctrl Pts',(-22.7130842691032,-70.8071619049747,
85.3499706788249));
#178202=CARTESIAN_POINT('Ctrl Pts',(-22.7223276789988,-70.4152854548392,
85.2099616521215));
#178203=CARTESIAN_POINT('Ctrl Pts',(-22.7506180336334,-69.2331495062128,
84.7227331440658));
#178204=CARTESIAN_POINT('Ctrl Pts',(-22.7693292570255,-68.4700986548075,
84.3156960176756));
#178205=CARTESIAN_POINT('Ctrl Pts',(-22.8052308235053,-67.1177286366594,
83.4119184043845));
#178206=CARTESIAN_POINT('Ctrl Pts',(-22.8222017284822,-66.5211288698208,
82.9325431138843));
#178207=CARTESIAN_POINT('Ctrl Pts',(-22.8480288852443,-65.6699239372478,
82.1159758633101));
#178208=CARTESIAN_POINT('Ctrl Pts',(-22.8571021742464,-65.3838726097524,
81.8140391787974));
#178209=CARTESIAN_POINT('Ctrl Pts',(-22.8833462494765,-64.6039940379515,
80.9078298739082));
#178210=CARTESIAN_POINT('Ctrl Pts',(-22.9006651616273,-64.1492881082466,
80.2722764235936));
#178211=CARTESIAN_POINT('Ctrl Pts',(-22.9322238148094,-63.420985671439,
79.0333195354624));
#178212=CARTESIAN_POINT('Ctrl Pts',(-22.9464765218011,-63.1311932840505,
78.4423425760535));
#178213=CARTESIAN_POINT('Ctrl Pts',(-22.9770326934869,-62.6142163608826,
77.1494521765591));
#178214=CARTESIAN_POINT('Ctrl Pts',(-22.9933345129949,-62.3994438891434,
76.4450044857766));
#178215=CARTESIAN_POINT('Ctrl Pts',(-23.0260362176216,-62.0858017418872,
74.9840266933657));
#178216=CARTESIAN_POINT('Ctrl Pts',(-23.0424688984152,-61.9915363368737,
74.2293314714673));
#178217=CARTESIAN_POINT('Ctrl Pts',(-23.0769262950679,-61.9334218436445,
72.6616294686187));
#178218=CARTESIAN_POINT('Ctrl Pts',(-23.0947623215829,-61.9788001263085,
71.8514825686357));
#178219=CARTESIAN_POINT('Ctrl Pts',(-23.1306635972023,-62.2237507322968,
70.2192800241415));
#178220=CARTESIAN_POINT('Ctrl Pts',(-23.1490078637108,-62.4286147657149,
69.4017833384164));
#178221=CARTESIAN_POINT('Ctrl Pts',(-23.186048784348,-62.9937640693951,
67.8148486279439));
#178222=CARTESIAN_POINT('Ctrl Pts',(-23.2042716490927,-63.3532618081069,
67.0493206846451));
#178223=CARTESIAN_POINT('Ctrl Pts',(-23.2415311394046,-64.2262368425864,
65.5795356979476));
#178224=CARTESIAN_POINT('Ctrl Pts',(-23.2606445669586,-64.7413162631444,
64.8810382503422));
#178225=CARTESIAN_POINT('Ctrl Pts',(-23.2916628434666,-65.6972847449895,
63.8231523380311));
#178226=CARTESIAN_POINT('Ctrl Pts',(-23.3037627027081,-66.0991769513896,
63.4322008835633));
#178227=CARTESIAN_POINT('Ctrl Pts',(-23.3315230797198,-67.0667774133513,
62.605159897377));
#178228=CARTESIAN_POINT('Ctrl Pts',(-23.3472354467346,-67.6456480225656,
62.1872116077931));
#178229=CARTESIAN_POINT('Ctrl Pts',(-23.3770439007649,-68.815519792736,
61.480456318847));
#178230=CARTESIAN_POINT('Ctrl Pts',(-23.3911310382946,-69.3999296712872,
61.184839910032));
#178231=CARTESIAN_POINT('Ctrl Pts',(-23.4206027246984,-70.648251547133,
60.6670916472714));
#178232=CARTESIAN_POINT('Ctrl Pts',(-23.4359727849947,-71.3128536017084,
60.4519777741411));
#178233=CARTESIAN_POINT('Ctrl Pts',(-23.4668095013143,-72.6881582521576,
60.1257463559955));
#178234=CARTESIAN_POINT('Ctrl Pts',(-23.4822248385575,-73.3972883002128,
60.0181098992289));
#178235=CARTESIAN_POINT('Ctrl Pts',(-23.5043649020229,-74.40848676433,59.9488656461147));
#178236=CARTESIAN_POINT('Ctrl Pts',(-23.5108840566336,-74.7058106598718,
59.9387052680259));
#178237=CARTESIAN_POINT('Ctrl Pts',(-23.5174110875174,-75.0031087425464,
59.9387052680259));
#178238=CARTESIAN_POINT('Ctrl Pts',(-23.2177969711981,-75.0031087425464,
59.9387052680259));
#178239=CARTESIAN_POINT('Ctrl Pts',(-23.2123696959067,-74.7558473929478,
59.9387052680259));
#178240=CARTESIAN_POINT('Ctrl Pts',(-23.2069356605294,-74.5085120342089,
59.9457333592563));
#178241=CARTESIAN_POINT('Ctrl Pts',(-23.1870440719356,-73.6072176795643,
59.997047349715));
#178242=CARTESIAN_POINT('Ctrl Pts',(-23.1724726631029,-72.9567675916252,
60.0835149849251));
#178243=CARTESIAN_POINT('Ctrl Pts',(-23.1387649040543,-71.4692304011195,
60.3966045566484));
#178244=CARTESIAN_POINT('Ctrl Pts',(-23.1199621028945,-70.6426901946818,
60.6584441188451));
#178245=CARTESIAN_POINT('Ctrl Pts',(-23.0821642900146,-69.0734071685228,
61.3332941733369));
#178246=CARTESIAN_POINT('Ctrl Pts',(-23.0633856665419,-68.3327795084699,
61.7407906439637));
#178247=CARTESIAN_POINT('Ctrl Pts',(-23.0262799044402,-66.9385082822665,
62.6944000048576));
#178248=CARTESIAN_POINT('Ctrl Pts',(-23.0076587848129,-66.2884283456319,
63.2386606339165));
#178249=CARTESIAN_POINT('Ctrl Pts',(-22.9696489429302,-65.089360746866,
64.4589854659968));
#178250=CARTESIAN_POINT('Ctrl Pts',(-22.950760136218,-64.5459609327155,
65.1347407662965));
#178251=CARTESIAN_POINT('Ctrl Pts',(-22.9155386888329,-63.6726496477427,
66.4738119744188));
#178252=CARTESIAN_POINT('Ctrl Pts',(-22.8992021686245,-63.3244079052054,
67.1210541591254));
#178253=CARTESIAN_POINT('Ctrl Pts',(-22.8668711397119,-62.7420991952012,
68.4633079657042));
#178254=CARTESIAN_POINT('Ctrl Pts',(-22.8510088435519,-62.5084099403389,
69.1556632672244));
#178255=CARTESIAN_POINT('Ctrl Pts',(-22.8206476946401,-62.1788908517869,
70.4922565068026));
#178256=CARTESIAN_POINT('Ctrl Pts',(-22.8062474186823,-62.070940327118,
71.1312576104667));
#178257=CARTESIAN_POINT('Ctrl Pts',(-22.7751127380341,-61.9398092071712,
72.5372511441418));
#178258=CARTESIAN_POINT('Ctrl Pts',(-22.758505876112,-61.9358845560748,
73.303654728887));
#178259=CARTESIAN_POINT('Ctrl Pts',(-22.7324455406655,-62.0336043832685,
74.4817778955585));
#178260=CARTESIAN_POINT('Ctrl Pts',(-22.7232053297365,-62.0880162647817,
74.8956863581744));
#178261=CARTESIAN_POINT('Ctrl Pts',(-22.6948421594479,-62.3159267091236,
76.1577337341884));
#178262=CARTESIAN_POINT('Ctrl Pts',(-22.6760964756324,-62.553997005025,
76.9917910798007));
#178263=CARTESIAN_POINT('Ctrl Pts',(-22.6424505830227,-63.118420781376,
78.415564530002));
#178264=CARTESIAN_POINT('Ctrl Pts',(-22.6276767664198,-63.4110696739612,
79.0152810730968));
#178265=CARTESIAN_POINT('Ctrl Pts',(-22.5964536780277,-64.130251562773,
80.2411962973343));
#178266=CARTESIAN_POINT('Ctrl Pts',(-22.5801252206438,-64.5680610345939,
80.8579979938936));
#178267=CARTESIAN_POINT('Ctrl Pts',(-22.5543744219634,-65.3272491916067,
81.7520377711469));
#178268=CARTESIAN_POINT('Ctrl Pts',(-22.5451559795505,-65.6129093885819,
82.057419901823));
#178269=CARTESIAN_POINT('Ctrl Pts',(-22.516919888215,-66.5322453940485,
82.9501584093053));
#178270=CARTESIAN_POINT('Ctrl Pts',(-22.4982769191142,-67.2099523810732,
83.4887688967499));
#178271=CARTESIAN_POINT('Ctrl Pts',(-22.4640738082773,-68.5240941504044,
84.3354497482744));
#178272=CARTESIAN_POINT('Ctrl Pts',(-22.4486093883778,-69.1418384806561,
84.6664984142158));
#178273=CARTESIAN_POINT('Ctrl Pts',(-22.4165167298404,-70.4869128356522,
85.2536056933848));
#178274=CARTESIAN_POINT('Ctrl Pts',(-22.3999604916125,-71.2164354828224,
85.4980721619425));
#178275=CARTESIAN_POINT('Ctrl Pts',(-22.3720627248218,-72.4554404905535,
85.7948858721622));
#178276=CARTESIAN_POINT('Ctrl Pts',(-22.360913397835,-72.9541153397416,
85.8840633147286));
#178277=CARTESIAN_POINT('Ctrl Pts',(-22.3309591565491,-74.3117424637426,
86.0460983856683));
#178278=CARTESIAN_POINT('Ctrl Pts',(-22.3124587905585,-75.1747837319727,
86.0632601490741));
#178279=CARTESIAN_POINT('Ctrl Pts',(-22.2845439381383,-76.4467593173734,
85.9625327976298));
#178280=CARTESIAN_POINT('Ctrl Pts',(-22.2754261188661,-76.8585189587835,
85.910079867448));
#178281=CARTESIAN_POINT('Ctrl Pts',(-22.2479497859112,-78.0923377446237,
85.6927129397798));
#178282=CARTESIAN_POINT('Ctrl Pts',(-22.2299384351025,-78.9016750433963,
85.4681657864787));
#178283=CARTESIAN_POINT('Ctrl Pts',(-22.1963630139692,-80.3383096775272,
84.9160778634896));
#178284=CARTESIAN_POINT('Ctrl Pts',(-22.1809075997859,-80.9714103559225,
84.6122494653766));
#178285=CARTESIAN_POINT('Ctrl Pts',(-22.1498865798407,-82.2007044815308,
83.8952952213165));
#178286=CARTESIAN_POINT('Ctrl Pts',(-22.1343394179012,-82.7931166020135,
83.4804158618099));
#178287=CARTESIAN_POINT('Ctrl Pts',(-22.0996873551722,-84.0123479757959,
82.4661369479483));
#178288=CARTESIAN_POINT('Ctrl Pts',(-22.080688351565,-84.6200189723064,
81.8489994871049));
#178289=CARTESIAN_POINT('Ctrl Pts',(-22.043690851755,-85.6900364840045,
80.5215557984812));
#178290=CARTESIAN_POINT('Ctrl Pts',(-22.0253834532474,-86.1533078349851,
79.817264122057));
#178291=CARTESIAN_POINT('Ctrl Pts',(-21.9883886554898,-86.9387141208914,
78.3276836433768));
#178292=CARTESIAN_POINT('Ctrl Pts',(-21.9701755051764,-87.2586859117162,
77.5457118574822));
#178293=CARTESIAN_POINT('Ctrl Pts',(-21.9329730465891,-87.7491604203139,
75.9115124136033));
#178294=CARTESIAN_POINT('Ctrl Pts',(-21.9138874461547,-87.9146567082245,
75.0620736225233));
#178295=CARTESIAN_POINT('Ctrl Pts',(-21.8832775743841,-88.045338634546,
73.6649069858103));
#178296=CARTESIAN_POINT('Ctrl Pts',(-21.8715817793504,-88.0622044875514,
73.12467336566));
#178297=CARTESIAN_POINT('Ctrl Pts',(-21.8449720591184,-88.0246676027813,
71.9080495797004));
#178298=CARTESIAN_POINT('Ctrl Pts',(-21.8300144490856,-87.9511175274875,
71.2337992547658));
#178299=CARTESIAN_POINT('Ctrl Pts',(-21.7936672920935,-87.6443580933324,
69.607775881084));
#178300=CARTESIAN_POINT('Ctrl Pts',(-21.7725828052433,-87.3557864236126,
68.6706321687396));
#178301=CARTESIAN_POINT('Ctrl Pts',(-21.741871450258,-86.7992517857775,
67.393518066754));
#178302=CARTESIAN_POINT('Ctrl Pts',(-21.7326758901293,-86.6151054813704,
67.0206528993441));
#178303=CARTESIAN_POINT('Ctrl Pts',(-21.7066756118522,-86.0413009332282,
65.9863438652782));
#178304=CARTESIAN_POINT('Ctrl Pts',(-21.690065426756,-85.6106812483756,
65.3496032144281));
#178305=CARTESIAN_POINT('Ctrl Pts',(-21.6585775345741,-84.7080001966367,
64.2396374698938));
#178306=CARTESIAN_POINT('Ctrl Pts',(-21.6438352746905,-84.2507237753405,
63.757561024057));
#178307=CARTESIAN_POINT('Ctrl Pts',(-21.6098769346781,-83.1041922799144,
62.7199745475537));
#178308=CARTESIAN_POINT('Ctrl Pts',(-21.59067854922,-82.3911786697216,62.1955487260731));
#178309=CARTESIAN_POINT('Ctrl Pts',(-21.5619309785478,-81.2723054333921,
61.5358252856643));
#178310=CARTESIAN_POINT('Ctrl Pts',(-21.5526917073905,-80.9040126423071,
61.3417681468817));
#178311=CARTESIAN_POINT('Ctrl Pts',(-21.5284782116718,-79.9091842943437,
60.8769115349169));
#178312=CARTESIAN_POINT('Ctrl Pts',(-21.5136425067296,-79.2696016194965,
60.6370732223613));
#178313=CARTESIAN_POINT('Ctrl Pts',(-21.4795996204699,-77.7857795419246,
60.2097487304598));
#178314=CARTESIAN_POINT('Ctrl Pts',(-21.4603866287851,-76.9357391930337,
60.0538549661469));
#178315=CARTESIAN_POINT('Ctrl Pts',(-21.4335870203312,-75.7194752094565,
59.9534586080836));
#178316=CARTESIAN_POINT('Ctrl Pts',(-21.425739200257,-75.3613555812664,
59.9387052678182));
#178317=CARTESIAN_POINT('Ctrl Pts',(-21.4178560137238,-75.0031087349823,
59.9387052680259));
#178318=CARTESIAN_POINT('Origin',(-23.90845228375,-75.0031087425464,72.9873550812444));
#178319=CARTESIAN_POINT('',(-19.6178714446467,-75.0031006318966,59.9387052680284));
#178320=CARTESIAN_POINT('',(-19.9173382169355,-75.0031141882852,59.9387052680271));
#178321=CARTESIAN_POINT('',(-23.90845228375,-75.0031087425464,59.9387052680259));
#178322=CARTESIAN_POINT('',(-19.417776314132,-66.6125912877755,62.9938945755099));
#178323=CARTESIAN_POINT('Ctrl Pts',(-19.6178714446467,-75.0031006318966,
59.9387052680284));
#178324=CARTESIAN_POINT('Ctrl Pts',(-19.6014685026439,-74.2607437617124,
59.9387057294552));
#178325=CARTESIAN_POINT('Ctrl Pts',(-19.5849037811272,-73.5197379909757,
60.0020567382727));
#178326=CARTESIAN_POINT('Ctrl Pts',(-19.5521553242651,-72.053177418037,
60.2546657056371));
#178327=CARTESIAN_POINT('Ctrl Pts',(-19.5358475432087,-71.3304102074453,
60.4440397486732));
#178328=CARTESIAN_POINT('Ctrl Pts',(-19.5024014277746,-69.9091738803646,
60.9498755753139));
#178329=CARTESIAN_POINT('Ctrl Pts',(-19.4854578253639,-69.2143639188463,
61.26816030853));
#178330=CARTESIAN_POINT('Ctrl Pts',(-19.4513770173664,-67.8656046389107,
62.0353827008749));
#178331=CARTESIAN_POINT('Ctrl Pts',(-19.4340082401172,-67.2166509500368,
62.4868441028642));
#178332=CARTESIAN_POINT('Ctrl Pts',(-19.4164777809729,-66.6124627542204,
62.9941412915471));
#178333=CARTESIAN_POINT('',(-19.7174312187883,-66.6129973379348,62.9934580993662));
#178334=CARTESIAN_POINT('Ctrl Pts',(-19.4175483972726,-66.6126744602016,
62.9939635397476));
#178335=CARTESIAN_POINT('Ctrl Pts',(-19.5175444259387,-66.6116381403926,
62.9948336320698));
#178336=CARTESIAN_POINT('Ctrl Pts',(-19.6175404546048,-66.6116382109846,
62.9948335017092));
#178337=CARTESIAN_POINT('Ctrl Pts',(-19.7175364832709,-66.6130192454567,
62.993674068783));
#178338=CARTESIAN_POINT('Ctrl Pts',(-19.9173382169355,-75.0031141882852,
59.9387052680271));
#178339=CARTESIAN_POINT('Ctrl Pts',(-19.9007967949276,-74.2445563629071,
59.9387049514496));
#178340=CARTESIAN_POINT('Ctrl Pts',(-19.8844783676533,-73.4874434635508,
60.0048502818403));
#178341=CARTESIAN_POINT('Ctrl Pts',(-19.8511771565402,-71.9905968512035,
60.2684072581934));
#178342=CARTESIAN_POINT('Ctrl Pts',(-19.8344745302453,-71.2538016732615,
60.4657909926964));
#178343=CARTESIAN_POINT('Ctrl Pts',(-19.8097614398516,-70.1848551286669,
60.8550310149607));
#178344=CARTESIAN_POINT('Ctrl Pts',(-19.8016215987501,-69.8370130284161,
60.9990145028378));
#178345=CARTESIAN_POINT('Ctrl Pts',(-19.7685609555398,-68.4584106326462,
61.640821849789));
#178346=CARTESIAN_POINT('Ctrl Pts',(-19.7433909837073,-67.4889730272299,
62.258205377191));
#178347=CARTESIAN_POINT('Ctrl Pts',(-19.7185673678502,-66.6125447149948,
62.9940724750352));
#178348=CARTESIAN_POINT('Origin',(-30.2175364832709,-75.,72.98888938658));
#178349=CARTESIAN_POINT('',(-21.9012048916249,-75.,85.23888938658));
#178350=CARTESIAN_POINT('',(-21.2338306941238,-75.,85.23888938658));
#178351=CARTESIAN_POINT('',(-30.2175364832709,-75.,85.23888938658));
#178352=CARTESIAN_POINT('',(-20.333830095635,-75.0000012548192,60.7388893865801));
#178353=CARTESIAN_POINT('Ctrl Pts',(-21.2338306941238,-75.,85.23888938658));
#178354=CARTESIAN_POINT('Ctrl Pts',(-21.2306064320489,-75.1377250058455,
85.23888938658));
#178355=CARTESIAN_POINT('Ctrl Pts',(-21.2273866755216,-75.2754746736316,
85.2365667529554));
#178356=CARTESIAN_POINT('Ctrl Pts',(-21.2078116035036,-76.1137341068034,
85.2082763223829));
#178357=CARTESIAN_POINT('Ctrl Pts',(-21.1916182257208,-76.810955591155,
85.1245500444249));
#178358=CARTESIAN_POINT('Ctrl Pts',(-21.1659705196501,-77.879673500507,
84.9020176777777));
#178359=CARTESIAN_POINT('Ctrl Pts',(-21.1567744412272,-78.2581393887295,
84.8041199660589));
#178360=CARTESIAN_POINT('Ctrl Pts',(-21.1286306389688,-79.4051451785294,
84.4481109454274));
#178361=CARTESIAN_POINT('Ctrl Pts',(-21.1099683881167,-80.1532725878486,
84.1317275942547));
#178362=CARTESIAN_POINT('Ctrl Pts',(-21.0785119861276,-81.3307116932154,
83.4896691172602));
#178363=CARTESIAN_POINT('Ctrl Pts',(-21.0660031776475,-81.7797483939057,
83.205508177142));
#178364=CARTESIAN_POINT('Ctrl Pts',(-21.0346129911703,-82.8643483604228,
82.4160666426164));
#178365=CARTESIAN_POINT('Ctrl Pts',(-21.0159325702271,-83.4707913209333,
81.8751337942049));
#178366=CARTESIAN_POINT('Ctrl Pts',(-20.9877251688978,-84.2833073570522,
80.9910685407017));
#178367=CARTESIAN_POINT('Ctrl Pts',(-20.978542572352,-84.5334034172025,
80.6914140839258));
#178368=CARTESIAN_POINT('Ctrl Pts',(-20.9504103312409,-85.2576446298438,
79.7342338652322));
#178369=CARTESIAN_POINT('Ctrl Pts',(-20.9317488399315,-85.6812092600103,
79.0412205812099));
#178370=CARTESIAN_POINT('Ctrl Pts',(-20.9008496550773,-86.2537312242886,
77.8544357222563));
#178371=CARTESIAN_POINT('Ctrl Pts',(-20.8888901159346,-86.4456055879746,
77.384127955797));
#178372=CARTESIAN_POINT('Ctrl Pts',(-20.8580282641812,-86.8667578848845,
76.1352399480246));
#178373=CARTESIAN_POINT('Ctrl Pts',(-20.8393588367127,-87.0488915854874,
75.3433905021401));
#178374=CARTESIAN_POINT('Ctrl Pts',(-20.8108520335845,-87.2025781778472,
74.1389171989822));
#178375=CARTESIAN_POINT('Ctrl Pts',(-20.8013448125835,-87.233848160121,
73.7361764964692));
#178376=CARTESIAN_POINT('Ctrl Pts',(-20.7728875543568,-87.2679058104121,
72.5229272900381));
#178377=CARTESIAN_POINT('Ctrl Pts',(-20.7542266297324,-87.2102682856516,
71.712966244044));
#178378=CARTESIAN_POINT('Ctrl Pts',(-20.7140962005733,-86.9203307398547,
70.0253900318385));
#178379=CARTESIAN_POINT('Ctrl Pts',(-20.6929048898017,-86.6697671416374,
69.1557229615675));
#178380=CARTESIAN_POINT('Ctrl Pts',(-20.6627410197266,-86.1756530420926,
67.9566977656067));
#178381=CARTESIAN_POINT('Ctrl Pts',(-20.653577681573,-86.0077871259066,
67.5993814610305));
#178382=CARTESIAN_POINT('Ctrl Pts',(-20.6321211873006,-85.5792460322651,
66.7910845979833));
#178383=CARTESIAN_POINT('Ctrl Pts',(-20.6198593184561,-85.306478951447,
66.3473741622852));
#178384=CARTESIAN_POINT('Ctrl Pts',(-20.5887064250236,-84.5387213002112,
65.2602169756139));
#178385=CARTESIAN_POINT('Ctrl Pts',(-20.570031460076,-84.0065472535975,
64.6461268255294));
#178386=CARTESIAN_POINT('Ctrl Pts',(-20.5418670051956,-83.1353033545976,
63.822082051671));
#178387=CARTESIAN_POINT('Ctrl Pts',(-20.5327174220962,-82.8404264015553,
63.5686329215459));
#178388=CARTESIAN_POINT('Ctrl Pts',(-20.5078304802431,-82.0034257913031,
62.9157914966793));
#178389=CARTESIAN_POINT('Ctrl Pts',(-20.4922564045862,-81.4396531612366,
62.5463734080976));
#178390=CARTESIAN_POINT('Ctrl Pts',(-20.4532579389303,-79.9700443453893,
61.7478730057183));
#178391=CARTESIAN_POINT('Ctrl Pts',(-20.4296832227902,-79.0365557338568,
61.3799267732218));
#178392=CARTESIAN_POINT('Ctrl Pts',(-20.3944895648947,-77.5721200205929,
61.0009833763027));
#178393=CARTESIAN_POINT('Ctrl Pts',(-20.3825725228186,-77.0678749125199,
60.9037917831714));
#178394=CARTESIAN_POINT('Ctrl Pts',(-20.358270691628,-76.0419975995413,
60.7721607017485));
#178395=CARTESIAN_POINT('Ctrl Pts',(-20.346008912442,-75.5212703996809,
60.7388894399758));
#178396=CARTESIAN_POINT('Ctrl Pts',(-20.333830095635,-75.0000012548192,
60.7388893865801));
#178397=CARTESIAN_POINT('',(-20.1338946865143,-67.1252798838891,63.6053345409727));
#178398=CARTESIAN_POINT('Ctrl Pts',(-20.333830095635,-75.0000012548192,
60.7388893865801));
#178399=CARTESIAN_POINT('Ctrl Pts',(-20.3171609122067,-74.2865385983972,
60.7388893134971));
#178400=CARTESIAN_POINT('Ctrl Pts',(-20.3006993175161,-73.5744403336657,
60.8012190536066));
#178401=CARTESIAN_POINT('Ctrl Pts',(-20.2672143173303,-72.1698753089757,
61.0489997289239));
#178402=CARTESIAN_POINT('Ctrl Pts',(-20.250461415262,-71.4800647066194,
61.2338634607188));
#178403=CARTESIAN_POINT('Ctrl Pts',(-20.2255958036809,-70.4769272751478,
61.5989754564678));
#178404=CARTESIAN_POINT('Ctrl Pts',(-20.2173661387531,-70.1490267795421,
61.7347175085119));
#178405=CARTESIAN_POINT('Ctrl Pts',(-20.1841011379601,-68.8555145895829,
62.3372463704191));
#178406=CARTESIAN_POINT('Ctrl Pts',(-20.1588428593053,-67.9471848925514,
62.9156573754958));
#178407=CARTESIAN_POINT('Ctrl Pts',(-20.1339068674138,-67.1258030253621,
63.6048858697113));
#178408=CARTESIAN_POINT('',(-19.4263813260168,-62.8761873158039,74.7426470661147));
#178409=CARTESIAN_POINT('Ctrl Pts',(-20.1339146423347,-67.1252326623533,
63.605364495691));
#178410=CARTESIAN_POINT('Ctrl Pts',(-20.0750070626096,-66.3344526705064,
64.2689966087264));
#178411=CARTESIAN_POINT('Ctrl Pts',(-20.0153558799609,-65.6307143557395,
65.0299429613649));
#178412=CARTESIAN_POINT('Ctrl Pts',(-19.8973223675187,-64.4233710241535,
66.7207259848254));
#178413=CARTESIAN_POINT('Ctrl Pts',(-19.8395215672342,-63.9273522053236,
67.6455451969498));
#178414=CARTESIAN_POINT('Ctrl Pts',(-19.7215871660935,-63.1867139032684,
69.5867095690456));
#178415=CARTESIAN_POINT('Ctrl Pts',(-19.6618458561676,-62.9420828473522,
70.5940527189565));
#178416=CARTESIAN_POINT('Ctrl Pts',(-19.5435268983665,-62.709918612146,
72.6588170657532));
#178417=CARTESIAN_POINT('Ctrl Pts',(-19.485538173564,-62.726548281685,73.7081850984939));
#178418=CARTESIAN_POINT('Ctrl Pts',(-19.4263813260168,-62.8761873158039,
74.7426470661147));
#178419=CARTESIAN_POINT('',(-19.1263815299174,-62.8761874826045,74.7426482192146));
#178420=CARTESIAN_POINT('',(-19.4263814899908,-62.8761746200905,74.7426467836703));
#178421=CARTESIAN_POINT('',(-19.0011490535824,-67.1252413014861,63.6053538167643));
#178422=CARTESIAN_POINT('Ctrl Pts',(-19.1263815299174,-62.8761874826045,
74.7426482192146));
#178423=CARTESIAN_POINT('Ctrl Pts',(-19.1161087162537,-62.7265520516628,
73.7082118549102));
#178424=CARTESIAN_POINT('Ctrl Pts',(-19.1067682656167,-62.7099182299581,
72.6588612733502));
#178425=CARTESIAN_POINT('Ctrl Pts',(-19.0856048538269,-62.9420706123676,
70.5941212219589));
#178426=CARTESIAN_POINT('Ctrl Pts',(-19.0740038291453,-63.1866916115569,
69.5867931485772));
#178427=CARTESIAN_POINT('Ctrl Pts',(-19.0533079901649,-63.9273116111903,
67.6456261303927));
#178428=CARTESIAN_POINT('Ctrl Pts',(-19.0441709589811,-64.4233323962465,
66.72078806223));
#178429=CARTESIAN_POINT('Ctrl Pts',(-19.02327760971,-65.6306771524171,65.0299871776315));
#178430=CARTESIAN_POINT('Ctrl Pts',(-19.0117355006677,-66.3344146039702,
64.2690330647641));
#178431=CARTESIAN_POINT('Ctrl Pts',(-19.0011200059672,-67.1252012611567,
63.6053908480438));
#178432=CARTESIAN_POINT('',(-19.2012431461282,-74.9999987591354,60.7388893865801));
#178433=CARTESIAN_POINT('Ctrl Pts',(-19.0011647644417,-67.1257997110858,
63.6048886507497));
#178434=CARTESIAN_POINT('Ctrl Pts',(-19.0263800941151,-67.9471805961339,
62.9156604862996));
#178435=CARTESIAN_POINT('Ctrl Pts',(-19.0510542001329,-68.8555096686468,
62.3372490326858));
#178436=CARTESIAN_POINT('Ctrl Pts',(-19.0845340441755,-70.1490234258174,
61.7347189482848));
#178437=CARTESIAN_POINT('Ctrl Pts',(-19.0928876791463,-70.4769239228417,
61.5989767903966));
#178438=CARTESIAN_POINT('Ctrl Pts',(-19.1179505022708,-71.4800592803612,
61.2338652070604));
#178439=CARTESIAN_POINT('Ctrl Pts',(-19.1344708541158,-72.1698680819012,
61.0490012011107));
#178440=CARTESIAN_POINT('Ctrl Pts',(-19.1676976678863,-73.5744386118425,
60.8012191599193));
#178441=CARTESIAN_POINT('Ctrl Pts',(-19.1845437886602,-74.2865381194436,
60.7388894588501));
#178442=CARTESIAN_POINT('Ctrl Pts',(-19.2012431461282,-74.9999987591354,
60.7388893865801));
#178443=CARTESIAN_POINT('',(-20.1012419544621,-75.,85.23888938658));
#178444=CARTESIAN_POINT('Ctrl Pts',(-19.2012431461282,-74.9999987591355,
60.7388893865801));
#178445=CARTESIAN_POINT('Ctrl Pts',(-19.2178347971233,-75.7088577649548,
60.7388893147761));
#178446=CARTESIAN_POINT('Ctrl Pts',(-19.2341852858951,-76.4163686749837,
60.8004162178675));
#178447=CARTESIAN_POINT('Ctrl Pts',(-19.2673328934291,-77.8106116762636,
61.0447571830811));
#178448=CARTESIAN_POINT('Ctrl Pts',(-19.2839937885109,-78.494782026441,
61.2267323451918));
#178449=CARTESIAN_POINT('Ctrl Pts',(-19.311244664781,-79.593309853432,61.6232931047021));
#178450=CARTESIAN_POINT('Ctrl Pts',(-19.3219325275506,-80.0179864860926,
61.8042979707288));
#178451=CARTESIAN_POINT('Ctrl Pts',(-19.3468572306141,-80.9759380243795,
62.2781617174915));
#178452=CARTESIAN_POINT('Ctrl Pts',(-19.3611960243164,-81.4996448467354,
62.5876329293234));
#178453=CARTESIAN_POINT('Ctrl Pts',(-19.3944166011216,-82.6628971902388,
63.3973133031375));
#178454=CARTESIAN_POINT('Ctrl Pts',(-19.413069929433,-83.280053766562,63.9247273598141));
#178455=CARTESIAN_POINT('Ctrl Pts',(-19.4412301671133,-84.1114166774393,
64.7914748368682));
#178456=CARTESIAN_POINT('Ctrl Pts',(-19.4504457623239,-84.3685202090294,
65.0865891827013));
#178457=CARTESIAN_POINT('Ctrl Pts',(-19.4759727466578,-85.0428155437503,
65.9398294921322));
#178458=CARTESIAN_POINT('Ctrl Pts',(-19.4921123752355,-85.4271994391204,
66.5219811776687));
#178459=CARTESIAN_POINT('Ctrl Pts',(-19.5272142319967,-86.1474679780081,
67.8455964083996));
#178460=CARTESIAN_POINT('Ctrl Pts',(-19.5463621687656,-86.4632789847727,
68.5942634992112));
#178461=CARTESIAN_POINT('Ctrl Pts',(-19.5772397965211,-86.8539719299969,
69.8572093570509));
#178462=CARTESIAN_POINT('Ctrl Pts',(-19.5890839114878,-86.974372130228,
70.3547896391956));
#178463=CARTESIAN_POINT('Ctrl Pts',(-19.6199096330926,-87.2042289723775,
71.6563126341651));
#178464=CARTESIAN_POINT('Ctrl Pts',(-19.6390505730574,-87.2656335795455,
72.4662047349187));
#178465=CARTESIAN_POINT('Ctrl Pts',(-19.6670600734787,-87.2374782401112,
73.6662943300324));
#178466=CARTESIAN_POINT('Ctrl Pts',(-19.6761146115089,-87.2096937876043,
74.0557205722193));
#178467=CARTESIAN_POINT('Ctrl Pts',(-19.7040719067252,-87.0671351656653,
75.2480705121353));
#178468=CARTESIAN_POINT('Ctrl Pts',(-19.7232146149536,-86.8912379171253,
76.0414467850986));
#178469=CARTESIAN_POINT('Ctrl Pts',(-19.7545879924084,-86.4723266558067,
77.3168214272262));
#178470=CARTESIAN_POINT('Ctrl Pts',(-19.7669023350968,-86.2736644264822,
77.8106903141346));
#178471=CARTESIAN_POINT('Ctrl Pts',(-19.7981973510168,-85.6928905608521,
79.0205688640787));
#178472=CARTESIAN_POINT('Ctrl Pts',(-19.8173406139994,-85.270624768396,
79.7144624313536));
#178473=CARTESIAN_POINT('Ctrl Pts',(-19.847486772466,-84.4931449152546,
80.7461161919661));
#178474=CARTESIAN_POINT('Ctrl Pts',(-19.8586396021926,-84.180915928759,
81.1132447328241));
#178475=CARTESIAN_POINT('Ctrl Pts',(-19.8887752040406,-83.2876110380681,
82.0461677596425));
#178476=CARTESIAN_POINT('Ctrl Pts',(-19.9079114798814,-82.6706680835386,
82.5742762522738));
#178477=CARTESIAN_POINT('Ctrl Pts',(-19.9377563186642,-81.6212087066361,
83.3059761542012));
#178478=CARTESIAN_POINT('Ctrl Pts',(-19.9486253805139,-81.2211899597887,
83.5520081760404));
#178479=CARTESIAN_POINT('Ctrl Pts',(-19.9784776666449,-80.0948208550819,
84.1585583275757));
#178480=CARTESIAN_POINT('Ctrl Pts',(-19.9976115130056,-79.3452541474879,
84.470939410336));
#178481=CARTESIAN_POINT('Ctrl Pts',(-20.0350217201929,-77.8110753435025,
84.9383825170732));
#178482=CARTESIAN_POINT('Ctrl Pts',(-20.0534076839674,-77.0311025355401,
85.0953814068152));
#178483=CARTESIAN_POINT('Ctrl Pts',(-20.0818291252186,-75.828729464966,
85.2178636174536));
#178484=CARTESIAN_POINT('Ctrl Pts',(-20.0915624256451,-75.4143798971417,
85.23888938658));
#178485=CARTESIAN_POINT('Ctrl Pts',(-20.1012419544621,-75.,85.23888938658));
#178486=CARTESIAN_POINT('',(-18.5675364832709,-75.,85.23888938658));
#178487=CARTESIAN_POINT('',(-30.2175364832709,-75.,85.23888938658));
#178488=CARTESIAN_POINT('Origin',(-18.5675364832709,-75.,72.98888938658));
#178489=CARTESIAN_POINT('Ctrl Pts',(-20.1012419544621,-75.,85.23888938658));
#178490=CARTESIAN_POINT('Ctrl Pts',(-20.1098579992633,-74.6311477731973,
85.23888938658));
#178491=CARTESIAN_POINT('Ctrl Pts',(-20.1184331195332,-74.2622715547378,
85.2222299412455));
#178492=CARTESIAN_POINT('Ctrl Pts',(-20.145877416015,-73.087224156511,85.115753719202));
#178493=CARTESIAN_POINT('Ctrl Pts',(-20.1649782572491,-72.2891976155929,
84.9626562940479));
#178494=CARTESIAN_POINT('Ctrl Pts',(-20.1977202056339,-70.9484151427787,
84.5644244052684));
#178495=CARTESIAN_POINT('Ctrl Pts',(-20.2113398668839,-70.3974549724233,
84.35660373583));
#178496=CARTESIAN_POINT('Ctrl Pts',(-20.2439365013652,-69.1278236305742,
83.7702075449523));
#178497=CARTESIAN_POINT('Ctrl Pts',(-20.2630835717669,-68.4276235773446,
83.3582260703368));
#178498=CARTESIAN_POINT('Ctrl Pts',(-20.2911519949849,-67.4567749344234,
82.6489038929779));
#178499=CARTESIAN_POINT('Ctrl Pts',(-20.3002500764559,-67.1515755586627,
82.4026218359583));
#178500=CARTESIAN_POINT('Ctrl Pts',(-20.3282394912505,-66.2529667088787,
81.6033603048994));
#178501=CARTESIAN_POINT('Ctrl Pts',(-20.3473742153681,-65.7022016462761,
81.0057866056215));
#178502=CARTESIAN_POINT('Ctrl Pts',(-20.3791352989799,-64.8850433499647,
79.9207080826668));
#178503=CARTESIAN_POINT('Ctrl Pts',(-20.3918182081102,-64.5852802091917,
79.4616066950045));
#178504=CARTESIAN_POINT('Ctrl Pts',(-20.4234809337223,-63.9206734423513,
78.2773350508884));
#178505=CARTESIAN_POINT('Ctrl Pts',(-20.4426256228864,-63.5951959624939,
77.5330701653992));
#178506=CARTESIAN_POINT('Ctrl Pts',(-20.4728580291676,-63.196193285558,
76.3006741841303));
#178507=CARTESIAN_POINT('Ctrl Pts',(-20.4840921895732,-63.0743287590611,
75.8307437016975));
#178508=CARTESIAN_POINT('Ctrl Pts',(-20.5143089920941,-62.8241808655607,
74.5599525780504));
#178509=CARTESIAN_POINT('Ctrl Pts',(-20.5334459048401,-62.7469506126223,
73.7515122717918));
#178510=CARTESIAN_POINT('Ctrl Pts',(-20.5708752753044,-62.7531722258421,
72.1470863459014));
#178511=CARTESIAN_POINT('Ctrl Pts',(-20.5892688834294,-62.8335003297472,
71.3549662903585));
#178512=CARTESIAN_POINT('Ctrl Pts',(-20.6336253435835,-63.2049955670995,
69.5056949374356));
#178513=CARTESIAN_POINT('Ctrl Pts',(-20.6587656706778,-63.5622215670142,
68.4687124396808));
#178514=CARTESIAN_POINT('Ctrl Pts',(-20.6935541827797,-64.2275848730086,
67.143332573469));
#178515=CARTESIAN_POINT('Ctrl Pts',(-20.7027671383237,-64.4196940867455,
66.802404984226));
#178516=CARTESIAN_POINT('Ctrl Pts',(-20.7301847934922,-65.0413334271389,
65.8131232904221));
#178517=CARTESIAN_POINT('Ctrl Pts',(-20.7481357032069,-65.5165846133254,
65.1958484834529));
#178518=CARTESIAN_POINT('Ctrl Pts',(-20.7846359035095,-66.5828894218892,
64.0540723966837));
#178519=CARTESIAN_POINT('Ctrl Pts',(-20.8031673576678,-67.1725813883994,
63.5331911230243));
#178520=CARTESIAN_POINT('Ctrl Pts',(-20.8399662375233,-68.4498940416262,
62.6068244322778));
#178521=CARTESIAN_POINT('Ctrl Pts',(-20.8583400584759,-69.1354236449765,
62.2047389495531));
#178522=CARTESIAN_POINT('Ctrl Pts',(-20.8953953203869,-70.5654543317576,
61.5429209378203));
#178523=CARTESIAN_POINT('Ctrl Pts',(-20.9136304218762,-71.3058177537415,
61.2829758193711));
#178524=CARTESIAN_POINT('Ctrl Pts',(-20.9491254009607,-72.7872992193625,
60.9174960981567));
#178525=CARTESIAN_POINT('Ctrl Pts',(-20.9666212717685,-73.5233888346176,
60.8055321609235));
#178526=CARTESIAN_POINT('Ctrl Pts',(-21.0030209867884,-75.0734559861661,
60.7123688138211));
#178527=CARTESIAN_POINT('Ctrl Pts',(-21.0216751093077,-75.8846719839338,
60.7440657022435));
#178528=CARTESIAN_POINT('Ctrl Pts',(-21.0498342314644,-77.0742678618884,
60.9094464154216));
#178529=CARTESIAN_POINT('Ctrl Pts',(-21.0590502488745,-77.4589289532811,
60.9818415273505));
#178530=CARTESIAN_POINT('Ctrl Pts',(-21.0846189366024,-78.5185179938907,
61.2343232499738));
#178531=CARTESIAN_POINT('Ctrl Pts',(-21.1007988461708,-79.1824981283792,
61.4538772995856));
#178532=CARTESIAN_POINT('Ctrl Pts',(-21.1359406362732,-80.569214644824,
62.0479865168428));
#178533=CARTESIAN_POINT('Ctrl Pts',(-21.155088545207,-81.280755162341,62.440353055518));
#178534=CARTESIAN_POINT('Ctrl Pts',(-21.1859723044965,-82.3697246124248,
63.1903442669647));
#178535=CARTESIAN_POINT('Ctrl Pts',(-21.197822228415,-82.7725401964285,
63.5066984326108));
#178536=CARTESIAN_POINT('Ctrl Pts',(-21.2189561588785,-83.4487388621008,
64.1098752124259));
#178537=CARTESIAN_POINT('Ctrl Pts',(-21.2282354324976,-83.7302342046026,
64.3865008010614));
#178538=CARTESIAN_POINT('Ctrl Pts',(-21.2586709516802,-84.6086355588132,
65.3373099039359));
#178539=CARTESIAN_POINT('Ctrl Pts',(-21.2794961590458,-85.1446657587784,
66.0636963168416));
#178540=CARTESIAN_POINT('Ctrl Pts',(-21.3194054798936,-86.002709791375,
67.542881664105));
#178541=CARTESIAN_POINT('Ctrl Pts',(-21.3385368832819,-86.3386537709364,
68.2821328961576));
#178542=CARTESIAN_POINT('Ctrl Pts',(-21.366845478053,-86.7290037998938,
69.4313695560812));
#178543=CARTESIAN_POINT('Ctrl Pts',(-21.3762087030407,-86.8398654341242,
69.8198100631227));
#178544=CARTESIAN_POINT('Ctrl Pts',(-21.40449699031,-87.1150137129048,71.0024597484276));
#178545=CARTESIAN_POINT('Ctrl Pts',(-21.4236452306662,-87.2198772616073,
71.8081875427081));
#178546=CARTESIAN_POINT('Ctrl Pts',(-21.4611946394842,-87.2685122063475,
73.4152996624451));
#178547=CARTESIAN_POINT('Ctrl Pts',(-21.4796157718967,-87.2147651333003,
74.2127061848986));
#178548=CARTESIAN_POINT('Ctrl Pts',(-21.5169717251508,-86.9540341921901,
75.7799416387219));
#178549=CARTESIAN_POINT('Ctrl Pts',(-21.5354562493324,-86.7487911403512,
76.5462509272946));
#178550=CARTESIAN_POINT('Ctrl Pts',(-21.5727085414766,-86.1867213661318,
78.0462026760087));
#178551=CARTESIAN_POINT('Ctrl Pts',(-21.591765904968,-85.8277814604079,
78.7749324589671));
#178552=CARTESIAN_POINT('Ctrl Pts',(-21.6253895591423,-85.0694528617131,
79.9930811898409));
#178553=CARTESIAN_POINT('Ctrl Pts',(-21.6398565408902,-84.6993106228171,
80.4972818176621));
#178554=CARTESIAN_POINT('Ctrl Pts',(-21.6732968651578,-83.7642286605803,
81.5858463747827));
#178555=CARTESIAN_POINT('Ctrl Pts',(-21.6924449246834,-83.1764068116068,
82.1467135255278));
#178556=CARTESIAN_POINT('Ctrl Pts',(-21.7205354724368,-82.2280368066412,
82.8869760443013));
#178557=CARTESIAN_POINT('Ctrl Pts',(-21.7296499241723,-81.9071202675885,
83.1135289069823));
#178558=CARTESIAN_POINT('Ctrl Pts',(-21.7576512820501,-80.8919033173423,
83.759459534353));
#178559=CARTESIAN_POINT('Ctrl Pts',(-21.776781865191,-80.1664152904246,
84.1256686992288));
#178560=CARTESIAN_POINT('Ctrl Pts',(-21.8142821899548,-78.6704209245698,
84.7029447245979));
#178561=CARTESIAN_POINT('Ctrl Pts',(-21.832561147153,-77.9047858153812,
84.9158881957529));
#178562=CARTESIAN_POINT('Ctrl Pts',(-21.8603682992152,-76.7391633025329,
85.1210973853699));
#178563=CARTESIAN_POINT('Ctrl Pts',(-21.8695647919879,-76.3513423178009,
85.1703931784277));
#178564=CARTESIAN_POINT('Ctrl Pts',(-21.8862470655318,-75.6416511975222,
85.2262883894837));
#178565=CARTESIAN_POINT('Ctrl Pts',(-21.8937367490427,-75.3207934997004,
85.23888938658));
#178566=CARTESIAN_POINT('Ctrl Pts',(-21.9012048916249,-75.,85.23888938658));
#178567=CARTESIAN_POINT('Origin',(-30.2175364832709,-75.,72.98888938658));
#178568=CARTESIAN_POINT('',(-23.7011390782975,-75.,85.23888938658));
#178569=CARTESIAN_POINT('',(-23.0338668482845,-75.,85.23888938658));
#178570=CARTESIAN_POINT('',(-30.2175364832709,-75.,85.23888938658));
#178571=CARTESIAN_POINT('Ctrl Pts',(-23.0338668482845,-75.,85.23888938658));
#178572=CARTESIAN_POINT('Ctrl Pts',(-23.0262998213682,-75.3221275290304,
85.23888938658));
#178573=CARTESIAN_POINT('Ctrl Pts',(-23.0187520574098,-75.6443192851186,
85.2261833347588));
#178574=CARTESIAN_POINT('Ctrl Pts',(-23.0021110631907,-76.3552153782709,
85.1699594113113));
#178575=CARTESIAN_POINT('Ctrl Pts',(-22.9930462891128,-76.7429128769076,
85.1205558194789));
#178576=CARTESIAN_POINT('Ctrl Pts',(-22.9655012593938,-77.9081622466141,
84.9150515089088));
#178577=CARTESIAN_POINT('Ctrl Pts',(-22.9467881084611,-78.6735358073442,
84.7019538959952));
#178578=CARTESIAN_POINT('Ctrl Pts',(-22.9092981855756,-80.1691910224016,
84.1243808155406));
#178579=CARTESIAN_POINT('Ctrl Pts',(-22.8906024098433,-80.8945872066577,
83.7579908032428));
#178580=CARTESIAN_POINT('Ctrl Pts',(-22.8623198133254,-81.909707671069,
83.1117662916684));
#178581=CARTESIAN_POINT('Ctrl Pts',(-22.8530808382852,-82.2306302407263,
82.8850848256554));
#178582=CARTESIAN_POINT('Ctrl Pts',(-22.824902106691,-83.178870787705,82.1445137654766));
#178583=CARTESIAN_POINT('Ctrl Pts',(-22.8062350344313,-83.7665466798045,
81.5834832571938));
#178584=CARTESIAN_POINT('Ctrl Pts',(-22.7724413254797,-84.704392308442,
80.4911044305202));
#178585=CARTESIAN_POINT('Ctrl Pts',(-22.7576307643293,-85.0768946777483,
79.9827909842042));
#178586=CARTESIAN_POINT('Ctrl Pts',(-22.7258675315935,-85.7946398020826,
78.8261839460199));
#178587=CARTESIAN_POINT('Ctrl Pts',(-22.7089460654834,-86.1240687535363,
78.1709110718784));
#178588=CARTESIAN_POINT('Ctrl Pts',(-22.6824840211798,-86.5377102969475,
77.1239567949714));
#178589=CARTESIAN_POINT('Ctrl Pts',(-22.6732223531819,-86.6646548218113,
76.7509859093388));
#178590=CARTESIAN_POINT('Ctrl Pts',(-22.6450265951199,-86.9973091154328,
75.5935185211075));
#178591=CARTESIAN_POINT('Ctrl Pts',(-22.6263550089459,-87.1433282171846,
74.7941866258295));
#178592=CARTESIAN_POINT('Ctrl Pts',(-22.5907447062317,-87.2668104205586,
73.2826552319992));
#178593=CARTESIAN_POINT('Ctrl Pts',(-22.5741527572156,-87.2633568713064,
72.575340754826));
#178594=CARTESIAN_POINT('Ctrl Pts',(-22.5485936965896,-87.1633383413165,
71.4826400741407));
#178595=CARTESIAN_POINT('Ctrl Pts',(-22.5395218894431,-87.1090271249557,
71.0949390303734));
#178596=CARTESIAN_POINT('Ctrl Pts',(-22.5114905391636,-86.8856144647397,
69.9146944208019));
#178597=CARTESIAN_POINT('Ctrl Pts',(-22.4923599986056,-86.6564182770519,
69.1357839382328));
#178598=CARTESIAN_POINT('Ctrl Pts',(-22.4558442370873,-86.0680835663841,
67.6850317512595));
#178599=CARTESIAN_POINT('Ctrl Pts',(-22.438354726871,-85.7199633126631,
67.0126227254432));
#178600=CARTESIAN_POINT('Ctrl Pts',(-22.4020820150213,-84.8873137300267,
65.7140760295469));
#178601=CARTESIAN_POINT('Ctrl Pts',(-22.3837133357845,-84.3996427845281,
65.0940426269605));
#178602=CARTESIAN_POINT('Ctrl Pts',(-22.3469081045789,-83.3062230582697,
63.9499714314866));
#178603=CARTESIAN_POINT('Ctrl Pts',(-22.3281933730792,-82.7018506065069,
63.4297644457954));
#178604=CARTESIAN_POINT('Ctrl Pts',(-22.2905622558381,-81.3887496671941,
62.5054296299141));
#178605=CARTESIAN_POINT('Ctrl Pts',(-22.2719000999076,-80.6815276224345,
62.1059075553095));
#178606=CARTESIAN_POINT('Ctrl Pts',(-22.2405052754543,-79.456667547083,
61.5661199666943));
#178607=CARTESIAN_POINT('Ctrl Pts',(-22.2280571681325,-78.9600030982355,
61.3845830934975));
#178608=CARTESIAN_POINT('Ctrl Pts',(-22.1967252800081,-77.6754119885708,
61.0071614945103));
#178609=CARTESIAN_POINT('Ctrl Pts',(-22.1780462749118,-76.8768863022691,
60.8564152130231));
#178610=CARTESIAN_POINT('Ctrl Pts',(-22.1498480449613,-75.6810554373594,
60.7516270575066));
#178611=CARTESIAN_POINT('Ctrl Pts',(-22.1406722760618,-75.291363291028,
60.7361536121109));
#178612=CARTESIAN_POINT('Ctrl Pts',(-22.1125459768857,-74.0914493532944,
60.7457925788283));
#178613=CARTESIAN_POINT('Ctrl Pts',(-22.0938847507034,-73.2839428084524,
60.8326551856262));
#178614=CARTESIAN_POINT('Ctrl Pts',(-22.063245005785,-72.0048933676573,
61.1003054905414));
#178615=CARTESIAN_POINT('Ctrl Pts',(-22.0515411627234,-71.5254756547257,
61.2314758584835));
#178616=CARTESIAN_POINT('Ctrl Pts',(-22.0209260472362,-70.2880648252244,
61.6523557925693));
#178617=CARTESIAN_POINT('Ctrl Pts',(-22.0022602890765,-69.5485755014501,
61.9888304199635));
#178618=CARTESIAN_POINT('Ctrl Pts',(-21.9690290795513,-68.3241280300276,
62.6999682773972));
#178619=CARTESIAN_POINT('Ctrl Pts',(-21.9547717612397,-67.8237715270789,
63.042487347291));
#178620=CARTESIAN_POINT('Ctrl Pts',(-21.9217104988849,-66.7178005343234,
63.9266360087504));
#178621=CARTESIAN_POINT('Ctrl Pts',(-21.9029757870737,-66.136578207952,
64.494243126718));
#178622=CARTESIAN_POINT('Ctrl Pts',(-21.8653891778259,-65.1091821708323,
65.7187331359601));
#178623=CARTESIAN_POINT('Ctrl Pts',(-21.8470031674235,-64.6621100433805,
66.3698646914459));
#178624=CARTESIAN_POINT('Ctrl Pts',(-21.8101616320894,-63.8953533310233,
67.75600756508));
#178625=CARTESIAN_POINT('Ctrl Pts',(-21.7914281262343,-63.5788434313785,
68.488511004103));
#178626=CARTESIAN_POINT('Ctrl Pts',(-21.7537889598953,-63.0880856771948,
70.0181228372959));
#178627=CARTESIAN_POINT('Ctrl Pts',(-21.7351258049263,-62.91769907343,70.8123875774607));
#178628=CARTESIAN_POINT('Ctrl Pts',(-21.7031420584741,-62.765088256904,
72.1671592343946));
#178629=CARTESIAN_POINT('Ctrl Pts',(-21.6901134131729,-62.7404674381057,
72.7202445362462));
#178630=CARTESIAN_POINT('Ctrl Pts',(-21.6582246746268,-62.7721055193404,
74.0835589830707));
#178631=CARTESIAN_POINT('Ctrl Pts',(-21.6395302786362,-62.8713194665633,
74.8901552818726));
#178632=CARTESIAN_POINT('Ctrl Pts',(-21.6112531073854,-63.135734420121,
76.0639095032712));
#178633=CARTESIAN_POINT('Ctrl Pts',(-21.6020182292371,-63.2403416970923,
76.4424359642614));
#178634=CARTESIAN_POINT('Ctrl Pts',(-21.5738426915193,-63.6160958930757,
77.5852015375517));
#178635=CARTESIAN_POINT('Ctrl Pts',(-21.5551762657695,-63.9450352018044,
78.3280944544134));
#178636=CARTESIAN_POINT('Ctrl Pts',(-21.5216559429986,-64.6497030909703,
79.5703354249273));
#178637=CARTESIAN_POINT('Ctrl Pts',(-21.5071141918457,-64.9946922910918,
80.0838101461263));
#178638=CARTESIAN_POINT('Ctrl Pts',(-21.4737845652494,-65.8782661389111,
81.205510704053));
#178639=CARTESIAN_POINT('Ctrl Pts',(-21.455041961911,-66.4415023030875,
81.7906510242567));
#178640=CARTESIAN_POINT('Ctrl Pts',(-21.417405567818,-67.660078510766,82.8282291929578));
#178641=CARTESIAN_POINT('Ctrl Pts',(-21.3989810463424,-68.3099656213873,
83.2811438588942));
#178642=CARTESIAN_POINT('Ctrl Pts',(-21.3620612013757,-69.6937755080575,
84.0587466666254));
#178643=CARTESIAN_POINT('Ctrl Pts',(-21.3432906153452,-70.4250670072927,
84.380453808053));
#178644=CARTESIAN_POINT('Ctrl Pts',(-21.3056407689123,-71.9525150275356,
84.8814166417609));
#178645=CARTESIAN_POINT('Ctrl Pts',(-21.2869740863415,-72.7457946001394,
85.0569433530397));
#178646=CARTESIAN_POINT('Ctrl Pts',(-21.2565786399345,-74.0317092661945,
85.2101695732384));
#178647=CARTESIAN_POINT('Ctrl Pts',(-21.2451685319971,-74.5157019649551,
85.23888938658));
#178648=CARTESIAN_POINT('Ctrl Pts',(-21.2338306941238,-75.,85.23888938658));
#178649=CARTESIAN_POINT('Ctrl Pts',(-21.9012048916249,-75.,85.23888938658));
#178650=CARTESIAN_POINT('Ctrl Pts',(-21.9125782707414,-74.5114573603728,
85.23888938658));
#178651=CARTESIAN_POINT('Ctrl Pts',(-21.9239044356528,-74.0230636781948,
85.2096639342135));
#178652=CARTESIAN_POINT('Ctrl Pts',(-21.9478457964892,-73.0096501981885,
85.087798589088));
#178653=CARTESIAN_POINT('Ctrl Pts',(-21.9603725158002,-72.4865450089706,
84.9900411043488));
#178654=CARTESIAN_POINT('Ctrl Pts',(-21.9917799006034,-71.1859644289943,
84.6581988150706));
#178655=CARTESIAN_POINT('Ctrl Pts',(-22.0104607484747,-70.4223137584041,
84.3803088616168));
#178656=CARTESIAN_POINT('Ctrl Pts',(-22.0386708144301,-69.3400888442793,
83.8599584523561));
#178657=CARTESIAN_POINT('Ctrl Pts',(-22.0478553964703,-68.9967264445139,
83.6741804109702));
#178658=CARTESIAN_POINT('Ctrl Pts',(-22.0759893549854,-67.9694339540432,
83.0531878838158));
#178659=CARTESIAN_POINT('Ctrl Pts',(-22.0946509382444,-67.3193440801203,
82.5662839438867));
#178660=CARTESIAN_POINT('Ctrl Pts',(-22.1256282833728,-66.3456250945475,
81.6736541886862));
#178661=CARTESIAN_POINT('Ctrl Pts',(-22.1376648627038,-65.9911004793198,
81.3053234731041));
#178662=CARTESIAN_POINT('Ctrl Pts',(-22.1686009432322,-65.1360879987814,
80.2979754269664));
#178663=CARTESIAN_POINT('Ctrl Pts',(-22.1872716604109,-64.6742010588965,
79.6294747767257));
#178664=CARTESIAN_POINT('Ctrl Pts',(-22.2225387722643,-63.9469199604427,
78.3152463805165));
#178665=CARTESIAN_POINT('Ctrl Pts',(-22.2387949208875,-63.6639320783142,
77.6829525209448));
#178666=CARTESIAN_POINT('Ctrl Pts',(-22.2640205862288,-63.306769682862,
76.6609265485124));
#178667=CARTESIAN_POINT('Ctrl Pts',(-22.2730903437162,-63.1954908104488,
76.2857142817879));
#178668=CARTESIAN_POINT('Ctrl Pts',(-22.3062121802276,-62.8573307832031,
74.9064206931231));
#178669=CARTESIAN_POINT('Ctrl Pts',(-22.3304595909478,-62.7392060524829,
73.8801134406065));
#178670=CARTESIAN_POINT('Ctrl Pts',(-22.3635705750701,-62.7552096258592,
72.4566520932503));
#178671=CARTESIAN_POINT('Ctrl Pts',(-22.3727336918797,-62.7787026048876,
72.062575462975));
#178672=CARTESIAN_POINT('Ctrl Pts',(-22.3941777178521,-62.8771211376457,
71.1535425627586));
#178673=CARTESIAN_POINT('Ctrl Pts',(-22.4064273726188,-62.9659068575163,
70.6408488965085));
#178674=CARTESIAN_POINT('Ctrl Pts',(-22.4375685235945,-63.2758137808868,
69.347044370216));
#178675=CARTESIAN_POINT('Ctrl Pts',(-22.4562432421102,-63.5424162842912,
68.579427704002));
#178676=CARTESIAN_POINT('Ctrl Pts',(-22.4843567532244,-64.0451923873106,
67.4930690325406));
#178677=CARTESIAN_POINT('Ctrl Pts',(-22.4934557790672,-64.2240147061549,
67.150225775991));
#178678=CARTESIAN_POINT('Ctrl Pts',(-22.5215089054144,-64.8268883784244,
66.1167412905581));
#178679=CARTESIAN_POINT('Ctrl Pts',(-22.5401698467046,-65.3034247356707,
65.4592781454081));
#178680=CARTESIAN_POINT('Ctrl Pts',(-22.5802146006489,-66.4381635310434,
64.1817854434283));
#178681=CARTESIAN_POINT('Ctrl Pts',(-22.6013239012438,-67.1071103148403,
63.5775965683758));
#178682=CARTESIAN_POINT('Ctrl Pts',(-22.6314002579322,-68.1559973975493,
62.821409300512));
#178683=CARTESIAN_POINT('Ctrl Pts',(-22.6405576459214,-68.4868433151611,
62.6063650022873));
#178684=CARTESIAN_POINT('Ctrl Pts',(-22.6616871474955,-69.2651501216567,
62.1523432814897));
#178685=CARTESIAN_POINT('Ctrl Pts',(-22.6736287675801,-69.7182351649998,
61.924432935029));
#178686=CARTESIAN_POINT('Ctrl Pts',(-22.7044733471793,-70.9293950006989,
61.4065912085476));
#178687=CARTESIAN_POINT('Ctrl Pts',(-22.7231424866878,-71.7044473564294,
61.1626986090622));
#178688=CARTESIAN_POINT('Ctrl Pts',(-22.7516484377097,-72.8930797710573,
60.9146870002823));
#178689=CARTESIAN_POINT('Ctrl Pts',(-22.7611557181722,-73.2921072485263,
60.8518148159533));
#178690=CARTESIAN_POINT('Ctrl Pts',(-22.7896132260569,-74.4988970480152,
60.7223695192334));
#178691=CARTESIAN_POINT('Ctrl Pts',(-22.8082741749799,-75.3108695269922,
60.7160750506029));
#178692=CARTESIAN_POINT('Ctrl Pts',(-22.848284711387,-77.0109977858797,
60.8718176690941));
#178693=CARTESIAN_POINT('Ctrl Pts',(-22.8693612475713,-77.8928146678276,
61.0515873940069));
#178694=CARTESIAN_POINT('Ctrl Pts',(-22.899402690759,-79.1224479328808,
61.4466458197849));
#178695=CARTESIAN_POINT('Ctrl Pts',(-22.9085577406908,-79.4917949500698,
61.5853048049218));
#178696=CARTESIAN_POINT('Ctrl Pts',(-22.9295606185864,-80.3141866489313,
61.9402090237461));
#178697=CARTESIAN_POINT('Ctrl Pts',(-22.9413782193905,-80.7619300973313,
62.1669634645486));
#178698=CARTESIAN_POINT('Ctrl Pts',(-22.9721031811024,-81.8937436046736,
62.8303613381045));
#178699=CARTESIAN_POINT('Ctrl Pts',(-22.9907704545007,-82.5505733677596,
63.3085880388868));
#178700=CARTESIAN_POINT('Ctrl Pts',(-23.0246481285778,-83.6275270917642,
64.2694450891077));
#178701=CARTESIAN_POINT('Ctrl Pts',(-23.0395412175759,-84.0663591901492,
64.7266821152755));
#178702=CARTESIAN_POINT('Ctrl Pts',(-23.0714953847188,-84.9353750704311,
65.785169794588));
#178703=CARTESIAN_POINT('Ctrl Pts',(-23.0885313434982,-85.350533922909,
66.3955822364597));
#178704=CARTESIAN_POINT('Ctrl Pts',(-23.115121820679,-85.8998462468878,
67.3843050696062));
#178705=CARTESIAN_POINT('Ctrl Pts',(-23.124395924343,-86.0746091169767,
67.7380754007731));
#178706=CARTESIAN_POINT('Ctrl Pts',(-23.152600459397,-86.5555332339301,
68.8428995309868));
#178707=CARTESIAN_POINT('Ctrl Pts',(-23.171275342588,-86.8044920144504,
69.6164202927912));
#178708=CARTESIAN_POINT('Ctrl Pts',(-23.1994228629323,-87.0569153815377,
70.7880363075798));
#178709=CARTESIAN_POINT('Ctrl Pts',(-23.2085556457866,-87.1205556841311,
71.1708978212189));
#178710=CARTESIAN_POINT('Ctrl Pts',(-23.2366418715287,-87.2606654242543,
72.3606066348551));
#178711=CARTESIAN_POINT('Ctrl Pts',(-23.2553027772918,-87.2753795146351,
73.1724963721619));
#178712=CARTESIAN_POINT('Ctrl Pts',(-23.2851263749657,-87.17244042403,74.4408006941545));
#178713=CARTESIAN_POINT('Ctrl Pts',(-23.2960263103336,-87.1089602337673,
74.8992388899376));
#178714=CARTESIAN_POINT('Ctrl Pts',(-23.3258610568216,-86.8633929460291,
76.1477690985458));
#178715=CARTESIAN_POINT('Ctrl Pts',(-23.3445220065786,-86.6286267135887,
76.9250870117486));
#178716=CARTESIAN_POINT('Ctrl Pts',(-23.3845289600388,-85.9758005354618,
78.5024246708648));
#178717=CARTESIAN_POINT('Ctrl Pts',(-23.4056020650923,-85.5427152277301,
79.2911461895476));
#178718=CARTESIAN_POINT('Ctrl Pts',(-23.4356398538035,-84.8009272233128,
80.3482224326073));
#178719=CARTESIAN_POINT('Ctrl Pts',(-23.4447946602598,-84.5589973564942,
80.6598428167345));
#178720=CARTESIAN_POINT('Ctrl Pts',(-23.46578440528,-83.9765759341496,81.3396051526625));
#178721=CARTESIAN_POINT('Ctrl Pts',(-23.4775891431064,-83.6276689178653,
81.6996126601055));
#178722=CARTESIAN_POINT('Ctrl Pts',(-23.508301690374,-82.6590475139244,
82.5835950680837));
#178723=CARTESIAN_POINT('Ctrl Pts',(-23.5269687829504,-82.0076454016134,
83.0691816056367));
#178724=CARTESIAN_POINT('Ctrl Pts',(-23.5607709951479,-80.7735138332313,
83.8113406047466));
#178725=CARTESIAN_POINT('Ctrl Pts',(-23.5755899146944,-80.2097333843237,
84.0937349816615));
#178726=CARTESIAN_POINT('Ctrl Pts',(-23.6073721691478,-78.9485792488077,
84.6081692691668));
#178727=CARTESIAN_POINT('Ctrl Pts',(-23.6243049028971,-78.2469636135959,
84.8234222667961));
#178728=CARTESIAN_POINT('Ctrl Pts',(-23.6507796690209,-77.1450156533659,
85.0560554886073));
#178729=CARTESIAN_POINT('Ctrl Pts',(-23.6600426239509,-76.7559946324765,
85.1187728869583));
#178730=CARTESIAN_POINT('Ctrl Pts',(-23.679943295204,-75.9112525200789,
85.2134651605353));
#178731=CARTESIAN_POINT('Ctrl Pts',(-23.6905408363261,-75.4556659020494,
85.23888938658));
#178732=CARTESIAN_POINT('Ctrl Pts',(-23.7011390782975,-75.,85.23888938658));
#178733=CARTESIAN_POINT('Origin',(-30.2175364832709,-75.,72.98888938658));
#178734=CARTESIAN_POINT('',(-25.5022222432624,-75.0000000426705,85.23888938658));
#178735=CARTESIAN_POINT('',(-24.8339325830033,-75.0000000321728,85.23888938658));
#178736=CARTESIAN_POINT('',(-30.2175364832709,-75.,85.23888938658));
#178737=CARTESIAN_POINT('Ctrl Pts',(-24.8339325837594,-75.0000000321906,
85.23888938658));
#178738=CARTESIAN_POINT('Ctrl Pts',(-24.8240890920827,-75.4186207774789,
85.23888938548));
#178739=CARTESIAN_POINT('Ctrl Pts',(-24.8142463699096,-75.8372234157294,
85.2174310040483));
#178740=CARTESIAN_POINT('Ctrl Pts',(-24.7917842720247,-76.7930051185784,
85.1190611901574));
#178741=CARTESIAN_POINT('Ctrl Pts',(-24.779240029544,-77.3275829231129,
85.0279214181392));
#178742=CARTESIAN_POINT('Ctrl Pts',(-24.7477156335147,-78.642378545885,
84.7128899054087));
#178743=CARTESIAN_POINT('Ctrl Pts',(-24.7285714438196,-79.4097119983233,
84.4463563610969));
#178744=CARTESIAN_POINT('Ctrl Pts',(-24.6983710047082,-80.5840955968139,
83.9028429934588));
#178745=CARTESIAN_POINT('Ctrl Pts',(-24.6871669947593,-81.0106812213281,
83.673842227766));
#178746=CARTESIAN_POINT('Ctrl Pts',(-24.6569802944016,-82.1124568073987,
82.9954752621748));
#178747=CARTESIAN_POINT('Ctrl Pts',(-24.6378436148025,-82.7584751441121,
82.503345126547));
#178748=CARTESIAN_POINT('Ctrl Pts',(-24.6079844560184,-83.6948921980658,
81.6307689182165));
#178749=CARTESIAN_POINT('Ctrl Pts',(-24.5971019203464,-84.019905075365,
81.2909700641096));
#178750=CARTESIAN_POINT('Ctrl Pts',(-24.5672361820081,-84.8499465114587,
80.3167309303754));
#178751=CARTESIAN_POINT('Ctrl Pts',(-24.5481022126914,-85.3128399117216,
79.6495232492781));
#178752=CARTESIAN_POINT('Ctrl Pts',(-24.5183347636273,-85.9329599516399,
78.5341685650817));
#178753=CARTESIAN_POINT('Ctrl Pts',(-24.5075385009762,-86.136010627728,
78.1142187159543));
#178754=CARTESIAN_POINT('Ctrl Pts',(-24.4777588966594,-86.6250909168048,
76.9355262006453));
#178755=CARTESIAN_POINT('Ctrl Pts',(-24.4586257282933,-86.8605662093157,
76.1583771809833));
#178756=CARTESIAN_POINT('Ctrl Pts',(-24.4212195702551,-87.1714573790356,
74.5851242120943));
#178757=CARTESIAN_POINT('Ctrl Pts',(-24.4028352669799,-87.2492868048642,
73.7934445278655));
#178758=CARTESIAN_POINT('Ctrl Pts',(-24.3586717168977,-87.2509629528297,
71.9154303363282));
#178759=CARTESIAN_POINT('Ctrl Pts',(-24.3337053505123,-87.1079379062421,
70.8356943427115));
#178760=CARTESIAN_POINT('Ctrl Pts',(-24.2990942202318,-86.7225084636294,
69.4114237720193));
#178761=CARTESIAN_POINT('Ctrl Pts',(-24.2898811077845,-86.6023221799552,
69.0390051751667));
#178762=CARTESIAN_POINT('Ctrl Pts',(-24.2624431493016,-86.190382005262,
67.9447527514958));
#178763=CARTESIAN_POINT('Ctrl Pts',(-24.2444727175805,-85.8474759337272,
67.2443071888604));
#178764=CARTESIAN_POINT('Ctrl Pts',(-24.2079540895495,-85.029865504896,
65.9121354125224));
#178765=CARTESIAN_POINT('Ctrl Pts',(-24.1894233646458,-84.5559184545767,
65.284145526537));
#178766=CARTESIAN_POINT('Ctrl Pts',(-24.1603876187993,-83.7140917278025,
64.3668975747821));
#178767=CARTESIAN_POINT('Ctrl Pts',(-24.1497308430971,-83.3841817416666,
64.045756103363));
#178768=CARTESIAN_POINT('Ctrl Pts',(-24.1200904967253,-82.42567845459,63.2124925373835));
#178769=CARTESIAN_POINT('Ctrl Pts',(-24.1009586935858,-81.7631562505982,
62.7429947730267));
#178770=CARTESIAN_POINT('Ctrl Pts',(-24.0726494833285,-80.7082953049164,
62.1426530032964));
#178771=CARTESIAN_POINT('Ctrl Pts',(-24.0632861415975,-80.3477750630805,
61.960436157542));
#178772=CARTESIAN_POINT('Ctrl Pts',(-24.0349981776565,-79.2383522775918,
61.4669175319571));
#178773=CARTESIAN_POINT('Ctrl Pts',(-24.0158499568544,-78.4669173928705,
61.2117952476941));
#178774=CARTESIAN_POINT('Ctrl Pts',(-23.9782996418965,-76.8978858706879,
60.8605644697829));
#178775=CARTESIAN_POINT('Ctrl Pts',(-23.9598787486126,-76.1046638010944,
60.7627717972648));
#178776=CARTESIAN_POINT('Ctrl Pts',(-23.9225209070743,-74.5163021095262,
60.7228769149453));
#178777=CARTESIAN_POINT('Ctrl Pts',(-23.9040340644223,-73.724947833655,
60.7797421661867));
#178778=CARTESIAN_POINT('Ctrl Pts',(-23.867818555596,-72.1897988286059,
61.0410216104658));
#178779=CARTESIAN_POINT('Ctrl Pts',(-23.8498266245349,-71.4486738007521,
61.2399809173404));
#178780=CARTESIAN_POINT('Ctrl Pts',(-23.816353900739,-70.1109997955915,
61.7373249692391));
#178781=CARTESIAN_POINT('Ctrl Pts',(-23.801028173916,-69.510696748442,62.0176736513018));
#178782=CARTESIAN_POINT('Ctrl Pts',(-23.7667340773171,-68.2317222814234,
62.7463376623581));
#178783=CARTESIAN_POINT('Ctrl Pts',(-23.7475858108103,-67.5690325328267,
63.2164706046294));
#178784=CARTESIAN_POINT('Ctrl Pts',(-23.7168375815155,-66.5758610383385,
64.0808839610502));
#178785=CARTESIAN_POINT('Ctrl Pts',(-23.7051159936441,-66.2150360684201,
64.4365162843896));
#178786=CARTESIAN_POINT('Ctrl Pts',(-23.6841121303596,-65.6140585796894,
65.1071305224153));
#178787=CARTESIAN_POINT('Ctrl Pts',(-23.6748340888881,-65.3652061057705,
65.4133522204306));
#178788=CARTESIAN_POINT('Ctrl Pts',(-23.6444357926001,-64.5991970897933,
66.4548887387677));
#178789=CARTESIAN_POINT('Ctrl Pts',(-23.6236457131505,-64.148089732302,
67.2351162176928));
#178790=CARTESIAN_POINT('Ctrl Pts',(-23.5837708328748,-63.4603125304579,
68.7991125321045));
#178791=CARTESIAN_POINT('Ctrl Pts',(-23.5646396113034,-63.2085878053367,
69.5711096082091));
#178792=CARTESIAN_POINT('Ctrl Pts',(-23.5272447654636,-62.8648131988296,
71.1371207779274));
#178793=CARTESIAN_POINT('Ctrl Pts',(-23.5088651754443,-62.7703863033566,
71.9266510474476));
#178794=CARTESIAN_POINT('Ctrl Pts',(-23.4717864698385,-62.7357437305451,
73.5030121464496));
#178795=CARTESIAN_POINT('Ctrl Pts',(-23.4535349993682,-62.7937115313033,
74.2861295015583));
#178796=CARTESIAN_POINT('Ctrl Pts',(-23.4164551921254,-63.0630028917562,
75.8572822715988));
#178797=CARTESIAN_POINT('Ctrl Pts',(-23.397351434627,-63.2789054964409,
76.6406718202847));
#178798=CARTESIAN_POINT('Ctrl Pts',(-23.3646755460105,-63.7812321879032,
77.9431193759609));
#178799=CARTESIAN_POINT('Ctrl Pts',(-23.3511192603518,-64.030745028914,
78.4734669276472));
#178800=CARTESIAN_POINT('Ctrl Pts',(-23.3185857738792,-64.7138240613626,
79.6906692077356));
#178801=CARTESIAN_POINT('Ctrl Pts',(-23.2994388168291,-65.1795868250031,
80.3563008656006));
#178802=CARTESIAN_POINT('Ctrl Pts',(-23.2690174517819,-66.0287446225397,
81.3448392015911));
#178803=CARTESIAN_POINT('Ctrl Pts',(-23.2576049321812,-66.3720958714854,
81.6989174992544));
#178804=CARTESIAN_POINT('Ctrl Pts',(-23.2272100597294,-67.3338647368048,
82.5779054743888));
#178805=CARTESIAN_POINT('Ctrl Pts',(-23.2080718369678,-67.9846391961632,
83.0637875831979));
#178806=CARTESIAN_POINT('Ctrl Pts',(-23.1800799565349,-69.0123713578003,
83.6829363660246));
#178807=CARTESIAN_POINT('Ctrl Pts',(-23.1710384235269,-69.3555489192395,
83.8679752644891));
#178808=CARTESIAN_POINT('Ctrl Pts',(-23.1430907969932,-70.4380163692609,
84.386605489894));
#178809=CARTESIAN_POINT('Ctrl Pts',(-23.123946444744,-71.2020358155108,
84.6634382317728));
#178810=CARTESIAN_POINT('Ctrl Pts',(-23.0926812947613,-72.4989119323465,
84.9924359645458));
#178811=CARTESIAN_POINT('Ctrl Pts',(-23.080469709526,-73.0178851199722,
85.0889634234049));
#178812=CARTESIAN_POINT('Ctrl Pts',(-23.0567980047726,-74.0257569555179,
85.2098250434086));
#178813=CARTESIAN_POINT('Ctrl Pts',(-23.045311437801,-74.5128050445081,
85.23888938658));
#178814=CARTESIAN_POINT('Ctrl Pts',(-23.0338668482845,-75.,85.23888938658));
#178815=CARTESIAN_POINT('',(-24.5016804832958,-70.810146674246,61.4773938111869));
#178816=CARTESIAN_POINT('Ctrl Pts',(-23.7011390782975,-75.,85.23888938658));
#178817=CARTESIAN_POINT('Ctrl Pts',(-23.7093709734307,-74.6460739496634,
85.23888938658));
#178818=CARTESIAN_POINT('Ctrl Pts',(-23.7176237986497,-74.2921005445638,
85.2235510126129));
#178819=CARTESIAN_POINT('Ctrl Pts',(-23.7426439198799,-73.2305729145749,
85.1312697475636));
#178820=CARTESIAN_POINT('Ctrl Pts',(-23.7593555478455,-72.5287710103631,
85.0080952031386));
#178821=CARTESIAN_POINT('Ctrl Pts',(-23.7850339826181,-71.4635413204302,
84.7238411137035));
#178822=CARTESIAN_POINT('Ctrl Pts',(-23.7941069531373,-71.0905026313075,
84.6048896260841));
#178823=CARTESIAN_POINT('Ctrl Pts',(-23.8216922606333,-69.9830109634707,
84.1923369604305));
#178824=CARTESIAN_POINT('Ctrl Pts',(-23.8403638222321,-69.2706713170174,
83.8453258300852));
#178825=CARTESIAN_POINT('Ctrl Pts',(-23.8760448608956,-67.9669247983626,
83.0459347916159));
#178826=CARTESIAN_POINT('Ctrl Pts',(-23.8931306014014,-67.3733273244117,
82.6035745495171));
#178827=CARTESIAN_POINT('Ctrl Pts',(-23.9197763709446,-66.5293923328939,
81.8470500810306));
#178828=CARTESIAN_POINT('Ctrl Pts',(-23.9290554590638,-66.2484678470804,
81.5696172793188));
#178829=CARTESIAN_POINT('Ctrl Pts',(-23.9572633824639,-65.4328354167441,
80.6823258149776));
#178830=CARTESIAN_POINT('Ctrl Pts',(-23.9759397936857,-64.9448372571729,
80.0325605683808));
#178831=CARTESIAN_POINT('Ctrl Pts',(-24.0041197058617,-64.32286214134,79.0065862565139));
#178832=CARTESIAN_POINT('Ctrl Pts',(-24.0132818683174,-64.1370893885365,
78.6643736992936));
#178833=CARTESIAN_POINT('Ctrl Pts',(-24.0413961707415,-63.6157767100914,
77.5843454866065));
#178834=CARTESIAN_POINT('Ctrl Pts',(-24.0600570986652,-63.3368680992437,
76.8216572022194));
#178835=CARTESIAN_POINT('Ctrl Pts',(-24.0902184752852,-63.0167121988657,
75.5754738617746));
#178836=CARTESIAN_POINT('Ctrl Pts',(-24.1014510015581,-62.9251664533932,
75.1073798151019));
#178837=CARTESIAN_POINT('Ctrl Pts',(-24.1316095233761,-62.7522382278562,
73.8322716919893));
#178838=CARTESIAN_POINT('Ctrl Pts',(-24.1502711001275,-62.7232758076924,
73.0205744395089));
#178839=CARTESIAN_POINT('Ctrl Pts',(-24.1812446426325,-62.8070419418149,
71.7024373076537));
#178840=CARTESIAN_POINT('Ctrl Pts',(-24.1932775224243,-62.871247683176,
71.1954139308815));
#178841=CARTESIAN_POINT('Ctrl Pts',(-24.2242100206175,-63.1187580708244,
69.8976782655188));
#178842=CARTESIAN_POINT('Ctrl Pts',(-24.2428806807743,-63.3492624146768,
69.1185135556219));
#178843=CARTESIAN_POINT('Ctrl Pts',(-24.2713913813562,-63.8073238446275,
67.9939421274307));
#178844=CARTESIAN_POINT('Ctrl Pts',(-24.2808987546529,-63.9780136014144,
67.6277967580806));
#178845=CARTESIAN_POINT('Ctrl Pts',(-24.3093553707275,-64.5445985287478,
66.5543506278136));
#178846=CARTESIAN_POINT('Ctrl Pts',(-24.3280161641349,-64.9928562708749,
65.8772242217274));
#178847=CARTESIAN_POINT('Ctrl Pts',(-24.3580370491845,-65.8020589964969,
64.8844487304048));
#178848=CARTESIAN_POINT('Ctrl Pts',(-24.3691318118908,-66.1202442711813,
64.5370247261621));
#178849=CARTESIAN_POINT('Ctrl Pts',(-24.4003010084835,-67.0732939630522,
63.6097814939158));
#178850=CARTESIAN_POINT('Ctrl Pts',(-24.4200738965064,-67.7502537057925,
63.0772037825501));
#178851=CARTESIAN_POINT('Ctrl Pts',(-24.4503832105327,-68.8430267947801,
62.3897936348474));
#178852=CARTESIAN_POINT('Ctrl Pts',(-24.4605586043277,-69.2206343750692,
62.1792601721665));
#178853=CARTESIAN_POINT('Ctrl Pts',(-24.4808914428694,-69.9997531482767,
61.7973829963986));
#178854=CARTESIAN_POINT('Ctrl Pts',(-24.4910333535345,-70.4008833660698,
61.6266532065697));
#178855=CARTESIAN_POINT('Ctrl Pts',(-24.5011646348533,-70.8102538861047,
61.4776545483405));
#178856=CARTESIAN_POINT('Ctrl Pts',(-24.5020520203782,-70.8102354594193,
61.477661255121));
#178857=CARTESIAN_POINT('Ctrl Pts',(-24.5170138898973,-71.4199016714757,
61.2557598343783));
#178858=CARTESIAN_POINT('Ctrl Pts',(-24.5316546309711,-72.0462294868208,
61.0826445498868));
#178859=CARTESIAN_POINT('Ctrl Pts',(-24.5602757693805,-73.2632244680831,
60.8482598525762));
#178860=CARTESIAN_POINT('Ctrl Pts',(-24.574394247675,-73.8504440319907,
60.7786574268127));
#178861=CARTESIAN_POINT('Ctrl Pts',(-24.607621744178,-75.2350038732028,
60.7153392574193));
#178862=CARTESIAN_POINT('Ctrl Pts',(-24.6264802640425,-76.0312995082613,
60.7564850607017));
#178863=CARTESIAN_POINT('Ctrl Pts',(-24.6563175955979,-77.3098798478237,
60.9483588610369));
#178864=CARTESIAN_POINT('Ctrl Pts',(-24.6676078796724,-77.7968319565327,
61.0520702099325));
#178865=CARTESIAN_POINT('Ctrl Pts',(-24.6863694883698,-78.5884181136076,
61.2717739860067));
#178866=CARTESIAN_POINT('Ctrl Pts',(-24.6937985887024,-78.8971436095272,
61.3708083634057));
#178867=CARTESIAN_POINT('Ctrl Pts',(-24.7389586259458,-80.7111991001541,
62.0331827774839));
#178868=CARTESIAN_POINT('Ctrl Pts',(-24.7776288169391,-82.0977571612455,
62.876148472946));
#178869=CARTESIAN_POINT('Ctrl Pts',(-24.8289724910095,-83.7555283971949,
64.3972525522298));
#178870=CARTESIAN_POINT('Ctrl Pts',(-24.8436758327869,-84.1941175156466,
64.8683164559407));
#178871=CARTESIAN_POINT('Ctrl Pts',(-24.8751693428624,-85.0173546005428,
65.9051592990021));
#178872=CARTESIAN_POINT('Ctrl Pts',(-24.8916156475598,-85.3957345879719,
66.4731130419377));
#178873=CARTESIAN_POINT('Ctrl Pts',(-24.9260540953204,-86.1004262191091,
67.7499114359243));
#178874=CARTESIAN_POINT('Ctrl Pts',(-24.9438298919491,-86.4103320355067,
68.4644349344013));
#178875=CARTESIAN_POINT('Ctrl Pts',(-24.9744933033455,-86.8256403399536,
69.7426445824062));
#178876=CARTESIAN_POINT('Ctrl Pts',(-24.9874728304087,-86.9631792015539,
70.2932967638212));
#178877=CARTESIAN_POINT('Ctrl Pts',(-25.0174918160325,-87.1839460707716,
71.5391680548982));
#178878=CARTESIAN_POINT('Ctrl Pts',(-25.0343743520946,-87.2467711270798,
72.2359985628576));
#178879=CARTESIAN_POINT('Ctrl Pts',(-25.069373645407,-87.2533583404747,
73.716367234393));
#178880=CARTESIAN_POINT('Ctrl Pts',(-25.0872874990229,-87.1819520576795,
74.4968924469779));
#178881=CARTESIAN_POINT('Ctrl Pts',(-25.1182337732407,-86.9299022857364,
75.8296327205571));
#178882=CARTESIAN_POINT('Ctrl Pts',(-25.1313641354787,-86.7836145760966,
76.3857733755451));
#178883=CARTESIAN_POINT('Ctrl Pts',(-25.1616235200426,-86.3730977679734,
77.5940615491839));
#178884=CARTESIAN_POINT('Ctrl Pts',(-25.1785926128937,-86.0906692279497,
78.237892470731));
#178885=CARTESIAN_POINT('Ctrl Pts',(-25.2137063690154,-85.3797439980679,
79.5414950453244));
#178886=CARTESIAN_POINT('Ctrl Pts',(-25.2316490835065,-84.9397667151215,
80.1914373133926));
#178887=CARTESIAN_POINT('Ctrl Pts',(-25.2636264458116,-84.046639685404,
81.2716017676295));
#178888=CARTESIAN_POINT('Ctrl Pts',(-25.2777934774843,-83.6169840088397,
81.7177314162769));
#178889=CARTESIAN_POINT('Ctrl Pts',(-25.3087673989437,-82.6450152742699,
82.5849394841047));
#178890=CARTESIAN_POINT('Ctrl Pts',(-25.3252836739824,-82.0973367114445,
82.9967993332136));
#178891=CARTESIAN_POINT('Ctrl Pts',(-25.3535589933042,-81.0836659351523,
83.6338335088741));
#178892=CARTESIAN_POINT('Ctrl Pts',(-25.3654650593838,-80.632456500941,
83.879310321471));
#178893=CARTESIAN_POINT('Ctrl Pts',(-25.3895534221763,-79.6802738010836,
84.3222881724379));
#178894=CARTESIAN_POINT('Ctrl Pts',(-25.4016967561352,-79.1790002497226,
84.516544952236));
#178895=CARTESIAN_POINT('Ctrl Pts',(-25.4219677213753,-78.3401187098178,
84.7796989058047));
#178896=CARTESIAN_POINT('Ctrl Pts',(-25.4299951547185,-78.009492109492,
84.8683899617203));
#178897=CARTESIAN_POINT('Ctrl Pts',(-25.4542801353021,-77.0137116115949,
85.0912648777087));
#178898=CARTESIAN_POINT('Ctrl Pts',(-25.470647235657,-76.340671534467,85.1841811302934));
#178899=CARTESIAN_POINT('Ctrl Pts',(-25.4918825248931,-75.4424234399546,
85.2328976122229));
#178900=CARTESIAN_POINT('Ctrl Pts',(-25.4970704667471,-75.2212078057676,
85.238889385809));
#178901=CARTESIAN_POINT('Ctrl Pts',(-25.5022222442556,-75.0000000426936,
85.23888938658));
#178902=CARTESIAN_POINT('Origin',(-30.2175364832709,-75.,72.98888938658));
#178903=CARTESIAN_POINT('',(-27.3010916068384,-75.,85.23888938658));
#178904=CARTESIAN_POINT('',(-26.6339799854461,-75.,85.23888938658));
#178905=CARTESIAN_POINT('',(-30.2175364832709,-75.,85.23888938658));
#178906=CARTESIAN_POINT('',(-25.633313136734,-70.8103134300187,61.4777794235982));
#178907=CARTESIAN_POINT('Ctrl Pts',(-26.6339799854461,-75.,85.23888938658));
#178908=CARTESIAN_POINT('Ctrl Pts',(-26.6191344608489,-75.6381113181522,
85.23888938658));
#178909=CARTESIAN_POINT('Ctrl Pts',(-26.6038014874433,-76.2753923550697,
85.1890298364595));
#178910=CARTESIAN_POINT('Ctrl Pts',(-26.55107738843,-78.4651155960251,84.8441233862049));
#178911=CARTESIAN_POINT('Ctrl Pts',(-26.5162064900661,-79.9621477761098,
84.2995345190604));
#178912=CARTESIAN_POINT('Ctrl Pts',(-26.4650951794551,-81.8044674005743,
83.1912670902666));
#178913=CARTESIAN_POINT('Ctrl Pts',(-26.4514103903528,-82.2730949941767,
82.8626618849234));
#178914=CARTESIAN_POINT('Ctrl Pts',(-26.4174837873031,-83.390798188754,
81.9560294276125));
#178915=CARTESIAN_POINT('Ctrl Pts',(-26.3977171030397,-84.0045770730602,
81.3394994348124));
#178916=CARTESIAN_POINT('Ctrl Pts',(-26.3402521639579,-85.5705161864811,
79.3912524177552));
#178917=CARTESIAN_POINT('Ctrl Pts',(-26.3007334647644,-86.328511742847,
77.9276020172795));
#178918=CARTESIAN_POINT('Ctrl Pts',(-26.2463389567453,-86.9800758096105,
75.6502720095092));
#178919=CARTESIAN_POINT('Ctrl Pts',(-26.2295436539528,-87.1184104644288,
74.9252011693067));
#178920=CARTESIAN_POINT('Ctrl Pts',(-26.1926456748223,-87.2711508562067,
73.3776538247701));
#178921=CARTESIAN_POINT('Ctrl Pts',(-26.173035722336,-87.2697165201255,
72.5571854533876));
#178922=CARTESIAN_POINT('Ctrl Pts',(-26.1356161371819,-87.1065512939891,
70.9611978811798));
#178923=CARTESIAN_POINT('Ctrl Pts',(-26.1178365702095,-86.9515753283765,
70.1888978228139));
#178924=CARTESIAN_POINT('Ctrl Pts',(-26.0845253654628,-86.5340109045882,
68.8107300735781));
#178925=CARTESIAN_POINT('Ctrl Pts',(-26.068876771263,-86.2944863433289,
68.2008865799041));
#178926=CARTESIAN_POINT('Ctrl Pts',(-26.0144120081656,-85.2910502638115,
66.1462570722396));
#178927=CARTESIAN_POINT('Ctrl Pts',(-25.9783338713947,-84.2886487783204,
64.8373035794661));
#178928=CARTESIAN_POINT('Ctrl Pts',(-25.9261162342618,-82.6338842686394,
63.3917374287345));
#178929=CARTESIAN_POINT('Ctrl Pts',(-25.9125953639996,-82.1833250516838,
63.0500080545254));
#178930=CARTESIAN_POINT('Ctrl Pts',(-25.8784056924184,-80.9705478192564,
62.2558564345393));
#178931=CARTESIAN_POINT('Ctrl Pts',(-25.8582495348373,-80.1799566242127,
61.8527550569305));
#178932=CARTESIAN_POINT('Ctrl Pts',(-25.8097366847142,-78.208345513547,
61.1032577663287));
#178933=CARTESIAN_POINT('Ctrl Pts',(-25.7800416048472,-77.0050537713077,
60.8422261194989));
#178934=CARTESIAN_POINT('Ctrl Pts',(-25.7334192216211,-75.0137007310833,
60.7146562684266));
#178935=CARTESIAN_POINT('Ctrl Pts',(-25.7159396638928,-74.2413171425731,
60.7381187694672));
#178936=CARTESIAN_POINT('Ctrl Pts',(-25.6770209109218,-72.5663055900796,
60.9480963661747));
#178937=CARTESIAN_POINT('Ctrl Pts',(-25.6549234401735,-71.672029307235,
61.1639951908746));
#178938=CARTESIAN_POINT('Ctrl Pts',(-25.6332414813969,-70.8102679226971,
61.4776494394493));
#178939=CARTESIAN_POINT('Ctrl Pts',(-25.6339066113238,-70.8102535523114,
61.4776546698313));
#178940=CARTESIAN_POINT('Ctrl Pts',(-25.6242937099174,-70.4261322987331,
61.6174633608416));
#178941=CARTESIAN_POINT('Ctrl Pts',(-25.6147024533179,-70.0492486347529,
61.7764115896691));
#178942=CARTESIAN_POINT('Ctrl Pts',(-25.5956768735074,-69.3152583045736,
62.1302028533648));
#178943=CARTESIAN_POINT('Ctrl Pts',(-25.5862533550733,-68.9584906670528,
62.3245785057338));
#178944=CARTESIAN_POINT('Ctrl Pts',(-25.5582468647041,-67.9316626967255,
62.9521117335403));
#178945=CARTESIAN_POINT('Ctrl Pts',(-25.5394278437801,-67.2935121541466,
63.4333497677411));
#178946=CARTESIAN_POINT('Ctrl Pts',(-25.5085183005986,-66.320848898401,
64.3280781054394));
#178947=CARTESIAN_POINT('Ctrl Pts',(-25.4963674127205,-65.9582084371738,
64.7073846238268));
#178948=CARTESIAN_POINT('Ctrl Pts',(-25.4652733071935,-65.0995746277491,
65.7293388705268));
#178949=CARTESIAN_POINT('Ctrl Pts',(-25.4461251728386,-64.641045296391,
66.4001451516963));
#178950=CARTESIAN_POINT('Ctrl Pts',(-25.415270760131,-64.0072048647155,
67.5591971914811));
#178951=CARTESIAN_POINT('Ctrl Pts',(-25.4034486513504,-63.7905065049081,
68.0219630866319));
#178952=CARTESIAN_POINT('Ctrl Pts',(-25.3726450418276,-63.3062091384989,
69.2506789863387));
#178953=CARTESIAN_POINT('Ctrl Pts',(-25.353504210212,-63.0846211875859,
70.0320819483146));
#178954=CARTESIAN_POINT('Ctrl Pts',(-25.3160474904702,-62.8016579372957,
71.6122576979627));
#178955=CARTESIAN_POINT('Ctrl Pts',(-25.297643697917,-62.7380386506744,
72.4066832473265));
#178956=CARTESIAN_POINT('Ctrl Pts',(-25.2604576408576,-62.7655029750708,
73.987755581599));
#178957=CARTESIAN_POINT('Ctrl Pts',(-25.2421276488185,-62.8548071581125,
74.7707279630282));
#178958=CARTESIAN_POINT('Ctrl Pts',(-25.2063268678832,-63.1753222669767,
76.2762133792397));
#178959=CARTESIAN_POINT('Ctrl Pts',(-25.1886072384691,-63.3996928090884,
76.9966778852067));
#178960=CARTESIAN_POINT('Ctrl Pts',(-25.1558679715698,-63.9358357907009,
78.2861385950576));
#178961=CARTESIAN_POINT('Ctrl Pts',(-25.1409607315228,-64.2293208450733,
78.8599241544918));
#178962=CARTESIAN_POINT('Ctrl Pts',(-25.1070825164293,-64.9912250232401,
80.0983083637154));
#178963=CARTESIAN_POINT('Ctrl Pts',(-25.0879342663996,-65.483397982614,
80.7447709155075));
#178964=CARTESIAN_POINT('Ctrl Pts',(-25.0598334224574,-66.3035771689732,
81.6253876379661));
#178965=CARTESIAN_POINT('Ctrl Pts',(-25.0507113522975,-66.5850369338083,
81.8998528009869));
#178966=CARTESIAN_POINT('Ctrl Pts',(-25.0227044718996,-67.4861461452905,
82.6977361539544));
#178967=CARTESIAN_POINT('Ctrl Pts',(-25.0035760654612,-68.1449440694906,
83.1735792585048));
#178968=CARTESIAN_POINT('Ctrl Pts',(-24.9715809479598,-69.3277697208447,
83.8608207678011));
#178969=CARTESIAN_POINT('Ctrl Pts',(-24.9586751843249,-69.8281865474364,
84.1075868446727));
#178970=CARTESIAN_POINT('Ctrl Pts',(-24.926790186775,-71.0931893099014,
84.6274461047887));
#178971=CARTESIAN_POINT('Ctrl Pts',(-24.9076447817233,-71.8714347608642,
84.8603362697242));
#178972=CARTESIAN_POINT('Ctrl Pts',(-24.8795977432193,-73.051108394981,
85.0891972153212));
#178973=CARTESIAN_POINT('Ctrl Pts',(-24.8705154761017,-73.4386120474841,
85.1452743685051));
#178974=CARTESIAN_POINT('Ctrl Pts',(-24.8522935929042,-74.2178734886321,
85.2201639890821));
#178975=CARTESIAN_POINT('Ctrl Pts',(-24.8431278920032,-74.6089450166963,
85.2388893876076));
#178976=CARTESIAN_POINT('Ctrl Pts',(-24.8339325837594,-75.0000000321906,
85.23888938658));
#178977=CARTESIAN_POINT('Ctrl Pts',(-25.5022222442556,-75.0000000426936,
85.23888938658));
#178978=CARTESIAN_POINT('Ctrl Pts',(-25.5084713324199,-74.7316757969748,
85.2388893875151));
#178979=CARTESIAN_POINT('Ctrl Pts',(-25.514666650198,-74.4633631194671,
85.2300733235928));
#178980=CARTESIAN_POINT('Ctrl Pts',(-25.5333912487406,-73.6492987417742,
85.1764949934327));
#178981=CARTESIAN_POINT('Ctrl Pts',(-25.5457654009036,-73.1061275916619,
85.1039777725178));
#178982=CARTESIAN_POINT('Ctrl Pts',(-25.5723880952531,-71.9740141827245,
84.8748141893723));
#178983=CARTESIAN_POINT('Ctrl Pts',(-25.5869006846059,-71.3882048389132,
84.7100966808637));
#178984=CARTESIAN_POINT('Ctrl Pts',(-25.6202442386018,-70.0801474247998,
84.2348780670153));
#178985=CARTESIAN_POINT('Ctrl Pts',(-25.6388269630157,-69.370629083816,
83.8970251730161));
#178986=CARTESIAN_POINT('Ctrl Pts',(-25.667453495464,-68.3075408310235,
83.2592888459669));
#178987=CARTESIAN_POINT('Ctrl Pts',(-25.6778214458911,-67.930189470185,
83.0032737999176));
#178988=CARTESIAN_POINT('Ctrl Pts',(-25.6994148362723,-67.1782982274196,
82.429428653647));
#178989=CARTESIAN_POINT('Ctrl Pts',(-25.710669108433,-66.8068287781899,
82.1089083842358));
#178990=CARTESIAN_POINT('Ctrl Pts',(-25.7390813344379,-65.947071862009,
81.2720365269247));
#178991=CARTESIAN_POINT('Ctrl Pts',(-25.7562503973109,-65.4825513593372,
80.7338373895999));
#178992=CARTESIAN_POINT('Ctrl Pts',(-25.7916170646537,-64.6076916526716,
79.5218014400891));
#178993=CARTESIAN_POINT('Ctrl Pts',(-25.809620682919,-64.2104203022293,
78.8424351649142));
#178994=CARTESIAN_POINT('Ctrl Pts',(-25.8418020885287,-63.618477832722,
77.5621262871115));
#178995=CARTESIAN_POINT('Ctrl Pts',(-25.8561163156436,-63.39990155571,76.9752736162829));
#178996=CARTESIAN_POINT('Ctrl Pts',(-25.8872534907432,-63.0380126342955,
75.7167863358488));
#178997=CARTESIAN_POINT('Ctrl Pts',(-25.9037721467167,-62.90435365929,75.044592911145));
#178998=CARTESIAN_POINT('Ctrl Pts',(-25.9320569832916,-62.7698421458036,
73.8545538722555));
#178999=CARTESIAN_POINT('Ctrl Pts',(-25.9439699925019,-62.7443072703597,
73.3412239802087));
#179000=CARTESIAN_POINT('Ctrl Pts',(-25.9680623120508,-62.7581191997014,
72.290953294684));
#179001=CARTESIAN_POINT('Ctrl Pts',(-25.9802029416912,-62.8004656078051,
71.7551487466587));
#179002=CARTESIAN_POINT('Ctrl Pts',(-26.000468032645,-62.9271055662463,
70.8853903304224));
#179003=CARTESIAN_POINT('Ctrl Pts',(-26.0084922369397,-62.9905403262234,
70.5491432531566));
#179004=CARTESIAN_POINT('Ctrl Pts',(-26.0327745664289,-63.2214967218882,
69.5553156321724));
#179005=CARTESIAN_POINT('Ctrl Pts',(-26.049142455272,-63.4296399047608,
68.9085279613618));
#179006=CARTESIAN_POINT('Ctrl Pts',(-26.0834613211641,-63.9882104728269,
67.5663054442032));
#179007=CARTESIAN_POINT('Ctrl Pts',(-26.1011950016354,-64.3534908965555,
66.8802249112739));
#179008=CARTESIAN_POINT('Ctrl Pts',(-26.1320399875461,-65.0989947316727,
65.7525420202517));
#179009=CARTESIAN_POINT('Ctrl Pts',(-26.1452507437363,-65.4503359376599,
65.2948302855941));
#179010=CARTESIAN_POINT('Ctrl Pts',(-26.1753704984884,-66.291534849655,
64.345749168081));
#179011=CARTESIAN_POINT('Ctrl Pts',(-26.192087918669,-66.793519764977,63.8677636821244));
#179012=CARTESIAN_POINT('Ctrl Pts',(-26.2268747712751,-67.9416175685551,
62.9464624790629));
#179013=CARTESIAN_POINT('Ctrl Pts',(-26.2447362273283,-68.5953162098822,
62.5174453487033));
#179014=CARTESIAN_POINT('Ctrl Pts',(-26.2756540367117,-69.7939413535712,
61.8852841361851));
#179015=CARTESIAN_POINT('Ctrl Pts',(-26.2888085887831,-70.3207606495648,
61.6532016257698));
#179016=CARTESIAN_POINT('Ctrl Pts',(-26.3190274266875,-71.5196809184391,
61.2229117616047));
#179017=CARTESIAN_POINT('Ctrl Pts',(-26.3359215262308,-72.1964195521106,
61.0435639041846));
#179018=CARTESIAN_POINT('Ctrl Pts',(-26.3694131377418,-73.5916853380126,
60.7989647952253));
#179019=CARTESIAN_POINT('Ctrl Pts',(-26.3859184135928,-74.308144060643,
60.737401243949));
#179020=CARTESIAN_POINT('Ctrl Pts',(-26.4177109943786,-75.7011732196679,
60.74034258804));
#179021=CARTESIAN_POINT('Ctrl Pts',(-26.4330985926661,-76.3751929350857,
60.7976060342426));
#179022=CARTESIAN_POINT('Ctrl Pts',(-26.4739857884841,-78.0711900623219,
61.0841949041665));
#179023=CARTESIAN_POINT('Ctrl Pts',(-26.499155897536,-79.0748638313095,
61.3893405302288));
#179024=CARTESIAN_POINT('Ctrl Pts',(-26.5394465847165,-80.6642260670412,
62.1046601011297));
#179025=CARTESIAN_POINT('Ctrl Pts',(-26.5551632226687,-81.2751974850627,
62.4450859704565));
#179026=CARTESIAN_POINT('Ctrl Pts',(-26.5845939189603,-82.3329564432275,
63.1591176833735));
#179027=CARTESIAN_POINT('Ctrl Pts',(-26.5983844180817,-82.7885729031909,
63.5160458859849));
#179028=CARTESIAN_POINT('Ctrl Pts',(-26.6309376155602,-83.7962167385299,
64.4274379540744));
#179029=CARTESIAN_POINT('Ctrl Pts',(-26.6494754220358,-84.3237927191043,
65.0052310096576));
#179030=CARTESIAN_POINT('Ctrl Pts',(-26.6835644303542,-85.2094407324633,
66.183687610807));
#179031=CARTESIAN_POINT('Ctrl Pts',(-26.6991835020518,-85.578253887105,
66.7724605973377));
#179032=CARTESIAN_POINT('Ctrl Pts',(-26.728358804406,-86.1570107765461,
67.898555466131));
#179033=CARTESIAN_POINT('Ctrl Pts',(-26.7419965753708,-86.3827231780006,
68.4255602597646));
#179034=CARTESIAN_POINT('Ctrl Pts',(-26.7742953617395,-86.8253937694119,
69.698908141503));
#179035=CARTESIAN_POINT('Ctrl Pts',(-26.792737966348,-87.0099148213698,
70.4539550779531));
#179036=CARTESIAN_POINT('Ctrl Pts',(-26.8263963701106,-87.2196775732373,
71.8925271405078));
#179037=CARTESIAN_POINT('Ctrl Pts',(-26.8416957334958,-87.2616311961265,
72.5706493668111));
#179038=CARTESIAN_POINT('Ctrl Pts',(-26.865152075445,-87.2399848251452,
73.5908530747913));
#179039=CARTESIAN_POINT('Ctrl Pts',(-26.8731285530494,-87.2183955747265,
73.9324971277993));
#179040=CARTESIAN_POINT('Ctrl Pts',(-26.8939927214038,-87.1262474567226,
74.8068612893775));
#179041=CARTESIAN_POINT('Ctrl Pts',(-26.9069422471566,-87.0349037508062,
75.3366528393326));
#179042=CARTESIAN_POINT('Ctrl Pts',(-26.93196383896,-86.788878395629,76.3575912142807));
#179043=CARTESIAN_POINT('Ctrl Pts',(-26.9440254854739,-86.6374386802978,
76.8484017458814));
#179044=CARTESIAN_POINT('Ctrl Pts',(-26.9717302316517,-86.2133448243849,
77.9679803642727));
#179045=CARTESIAN_POINT('Ctrl Pts',(-26.9871511958356,-85.9178672455006,
78.5862652773435));
#179046=CARTESIAN_POINT('Ctrl Pts',(-27.0172921810689,-85.256137022201,
79.7168904651298));
#179047=CARTESIAN_POINT('Ctrl Pts',(-27.0322121883741,-84.8990045324361,
80.2320943767446));
#179048=CARTESIAN_POINT('Ctrl Pts',(-27.0660250866552,-84.0086008696503,
81.3270148059124));
#179049=CARTESIAN_POINT('Ctrl Pts',(-27.0846480988713,-83.4556732047195,
81.8872515112947));
#179050=CARTESIAN_POINT('Ctrl Pts',(-27.119190643886,-82.3079336282323,
82.8459094481337));
#179051=CARTESIAN_POINT('Ctrl Pts',(-27.1351593915688,-81.7243938372151,
83.2528678063521));
#179052=CARTESIAN_POINT('Ctrl Pts',(-27.1628513724901,-80.6857202366822,
83.8504475038963));
#179053=CARTESIAN_POINT('Ctrl Pts',(-27.1744665975531,-80.2483714077816,
84.0683946597144));
#179054=CARTESIAN_POINT('Ctrl Pts',(-27.1970593913043,-79.3803882386793,
84.4379898624859));
#179055=CARTESIAN_POINT('Ctrl Pts',(-27.2079733236429,-78.9519631274399,
84.5928410494816));
#179056=CARTESIAN_POINT('Ctrl Pts',(-27.2375213755929,-77.7561380936208,
84.9511335733451));
#179057=CARTESIAN_POINT('Ctrl Pts',(-27.2557103241722,-76.976045372927,
85.1044514415865));
#179058=CARTESIAN_POINT('Ctrl Pts',(-27.2828493769064,-75.7921208368098,
85.219676211267));
#179059=CARTESIAN_POINT('Ctrl Pts',(-27.2918765948632,-75.396117741022,
85.23888938658));
#179060=CARTESIAN_POINT('Ctrl Pts',(-27.3010916068384,-75.,85.23888938658));
#179061=CARTESIAN_POINT('Origin',(-30.2175364832709,-75.,72.98888938658));
#179062=CARTESIAN_POINT('',(-28.5675339373409,-75.,85.23888938658));
#179063=CARTESIAN_POINT('',(-28.4332364523223,-75.,85.23888938658));
#179064=CARTESIAN_POINT('',(-30.2175364832709,-75.,85.23888938658));
#179065=CARTESIAN_POINT('',(-28.5670923992068,-69.49428841446,83.9313521779249));
#179066=CARTESIAN_POINT('Origin',(-28.5675339373409,-75.,72.98888938658));
#179067=CARTESIAN_POINT('Ctrl Pts',(-28.566799738496,-69.4940652583272,
83.9317949705847));
#179068=CARTESIAN_POINT('Ctrl Pts',(-28.5535796202282,-70.005706592258,
84.1892278593307));
#179069=CARTESIAN_POINT('Ctrl Pts',(-28.5405678519628,-70.5347700727441,
84.4104595782057));
#179070=CARTESIAN_POINT('Ctrl Pts',(-28.51473175451,-71.5927852950562,84.7680829344784));
#179071=CARTESIAN_POINT('Ctrl Pts',(-28.5017910892112,-72.1192331851877,
84.9077683006098));
#179072=CARTESIAN_POINT('Ctrl Pts',(-28.470017451143,-73.4269369811265,
85.163019254198));
#179073=CARTESIAN_POINT('Ctrl Pts',(-28.4514197440086,-74.2128528894147,
85.23888938658));
#179074=CARTESIAN_POINT('Ctrl Pts',(-28.4332364523223,-75.,85.23888938658));
#179075=CARTESIAN_POINT('Origin',(-30.2175364832709,-75.,72.98888938658));
#179076=CARTESIAN_POINT('',(-18.5675364832709,-75.,83.48888938658));
#179077=CARTESIAN_POINT('Origin',(-18.5675364832709,-75.,72.98888938658));
#179078=CARTESIAN_POINT('',(-16.5675364832709,-75.,83.48888938658));
#179079=CARTESIAN_POINT('',(-30.2175364832709,-75.,83.48888938658));
#179080=CARTESIAN_POINT('Origin',(-16.5675364832709,-75.,72.98888938658));
#179081=CARTESIAN_POINT('Origin',(-30.2175364832709,-75.,72.98888938658));
#179082=CARTESIAN_POINT('Ctrl Pts',(-28.4332364523223,-75.,85.23888938658));
#179083=CARTESIAN_POINT('Ctrl Pts',(-28.4272749810172,-75.2580696055256,
85.23888938658));
#179084=CARTESIAN_POINT('Ctrl Pts',(-28.4213453695568,-75.5162712590094,
85.2307343195952));
#179085=CARTESIAN_POINT('Ctrl Pts',(-28.4026862752731,-76.3283138333888,
85.1793092241826));
#179086=CARTESIAN_POINT('Ctrl Pts',(-28.3900005365992,-76.8793747916195,
85.1065915246954));
#179087=CARTESIAN_POINT('Ctrl Pts',(-28.3491296333933,-78.5779602068471,
84.7637573617779));
#179088=CARTESIAN_POINT('Ctrl Pts',(-28.3208970388223,-79.6927227764566,
84.3655227681864));
#179089=CARTESIAN_POINT('Ctrl Pts',(-28.2744393479831,-81.4747447009042,
83.4217145281043));
#179090=CARTESIAN_POINT('Ctrl Pts',(-28.2554501218592,-82.173743561816,
82.9540069009287));
#179091=CARTESIAN_POINT('Ctrl Pts',(-28.2169591966351,-83.4227685312124,
81.9182643494961));
#179092=CARTESIAN_POINT('Ctrl Pts',(-28.1981684404363,-83.9766830848617,
81.3612219855413));
#179093=CARTESIAN_POINT('Ctrl Pts',(-28.1616294311375,-84.9677267939973,
80.1523011524452));
#179094=CARTESIAN_POINT('Ctrl Pts',(-28.1439543387338,-85.4032183457479,
79.5037253200245));
#179095=CARTESIAN_POINT('Ctrl Pts',(-28.0882170797589,-86.5530413354272,
77.3785389502528));
#179096=CARTESIAN_POINT('Ctrl Pts',(-28.0486855424314,-87.035562094923,
75.7972772695498));
#179097=CARTESIAN_POINT('Ctrl Pts',(-27.998198245963,-87.2474686468745,
73.6060036740201));
#179098=CARTESIAN_POINT('Ctrl Pts',(-27.9852995732751,-87.2628958114621,
73.040908905797));
#179099=CARTESIAN_POINT('Ctrl Pts',(-27.9587146846565,-87.2157892732353,
71.9151151062079));
#179100=CARTESIAN_POINT('Ctrl Pts',(-27.9452213168172,-87.1536564102775,
71.3557522412607));
#179101=CARTESIAN_POINT('Ctrl Pts',(-27.9050939422032,-86.8517950145408,
69.6915179473661));
#179102=CARTESIAN_POINT('Ctrl Pts',(-27.8795411041813,-86.4975874087982,
68.6135998182178));
#179103=CARTESIAN_POINT('Ctrl Pts',(-27.8157427364997,-85.2837240160056,
66.1358619373885));
#179104=CARTESIAN_POINT('Ctrl Pts',(-27.7764672100201,-84.2817137597337,
64.8299194705179));
#179105=CARTESIAN_POINT('Ctrl Pts',(-27.7276820821519,-82.6784090297572,
63.431042310556));
#179106=CARTESIAN_POINT('Ctrl Pts',(-27.7162937230107,-82.2836321193268,
63.1268860837599));
#179107=CARTESIAN_POINT('Ctrl Pts',(-27.6857189744081,-81.2079789892142,
62.3980554752025));
#179108=CARTESIAN_POINT('Ctrl Pts',(-27.6664002680147,-80.5020014417848,
62.0147029161449));
#179109=CARTESIAN_POINT('Ctrl Pts',(-27.6273286349464,-78.9703639805918,
61.3682125268237));
#179110=CARTESIAN_POINT('Ctrl Pts',(-27.6077835078353,-78.1439873633118,
61.1179476012971));
#179111=CARTESIAN_POINT('Ctrl Pts',(-27.5502213684917,-75.690197005108,
60.6492701197406));
#179112=CARTESIAN_POINT('Ctrl Pts',(-27.510645118691,-74.0368111988532,
60.6675726774708));
#179113=CARTESIAN_POINT('Ctrl Pts',(-27.4593017697274,-71.8481262791416,
61.1360586866364));
#179114=CARTESIAN_POINT('Ctrl Pts',(-27.4455805910103,-71.2703427396734,
61.3049875462795));
#179115=CARTESIAN_POINT('Ctrl Pts',(-27.4042205380546,-69.6303259528372,
61.9185992688622));
#179116=CARTESIAN_POINT('Ctrl Pts',(-27.3766829939313,-68.6154260667505,
62.4711877981453));
#179117=CARTESIAN_POINT('Ctrl Pts',(-27.3306180247818,-67.0111323361636,
63.6635883552323));
#179118=CARTESIAN_POINT('Ctrl Pts',(-27.3114076338505,-66.3842576528396,
64.2394760263411));
#179119=CARTESIAN_POINT('Ctrl Pts',(-27.2666836146926,-65.1357009236572,
65.6518763485546));
#179120=CARTESIAN_POINT('Ctrl Pts',(-27.24195292677,-64.5506753257449,66.5121738831155));
#179121=CARTESIAN_POINT('Ctrl Pts',(-27.1972850869737,-63.6734096968681,
68.2371433892422));
#179122=CARTESIAN_POINT('Ctrl Pts',(-27.1769847565348,-63.3553270152619,
69.0809060502111));
#179123=CARTESIAN_POINT('Ctrl Pts',(-27.1369967096557,-62.9376635275748,
70.7129777021864));
#179124=CARTESIAN_POINT('Ctrl Pts',(-27.1181738246321,-62.8165549489823,
71.4910816820737));
#179125=CARTESIAN_POINT('Ctrl Pts',(-27.0815337674522,-62.7251842422228,
73.0571920400057));
#179126=CARTESIAN_POINT('Ctrl Pts',(-27.0637927592737,-62.7546442134893,
73.8415443202785));
#179127=CARTESIAN_POINT('Ctrl Pts',(-27.028524546933,-62.9577265860212,
75.3553303872461));
#179128=CARTESIAN_POINT('Ctrl Pts',(-27.0106861812567,-63.12369765144,76.0823979324076));
#179129=CARTESIAN_POINT('Ctrl Pts',(-26.9560904443609,-63.8360013351941,
78.2647375314558));
#179130=CARTESIAN_POINT('Ctrl Pts',(-26.9218022723306,-64.5932062142825,
79.6347969650691));
#179131=CARTESIAN_POINT('Ctrl Pts',(-26.8715478842229,-65.9470774062663,
81.2608741455193));
#179132=CARTESIAN_POINT('Ctrl Pts',(-26.858025490544,-66.3378175049943,
81.6691969574909));
#179133=CARTESIAN_POINT('Ctrl Pts',(-26.8233349394715,-67.424632085759,
82.6581833311752));
#179134=CARTESIAN_POINT('Ctrl Pts',(-26.8027190063633,-68.1593760086047,
83.1912081901998));
#179135=CARTESIAN_POINT('Ctrl Pts',(-26.7536317685482,-70.0151012546684,
84.2461241961342));
#179136=CARTESIAN_POINT('Ctrl Pts',(-26.7238224525624,-71.1695179694699,
84.6893982956736));
#179137=CARTESIAN_POINT('Ctrl Pts',(-26.676815145295,-73.1354002991896,
85.1214536861418));
#179138=CARTESIAN_POINT('Ctrl Pts',(-26.6590742007676,-73.9146647134644,
85.2158222533607));
#179139=CARTESIAN_POINT('Ctrl Pts',(-26.6386599166736,-74.7983961283731,
85.2376454334862));
#179140=CARTESIAN_POINT('Ctrl Pts',(-26.6363248807794,-74.899208394946,
85.23888938658));
#179141=CARTESIAN_POINT('Ctrl Pts',(-26.6339799854461,-75.,85.23888938658));
#179142=CARTESIAN_POINT('',(-28.2015531594526,-74.9999810209094,60.7388893865947));
#179143=CARTESIAN_POINT('Ctrl Pts',(-27.3010916068384,-75.,85.23888938658));
#179144=CARTESIAN_POINT('Ctrl Pts',(-27.305824079875,-74.796569279156,85.23888938658));
#179145=CARTESIAN_POINT('Ctrl Pts',(-27.3106166974195,-74.5931085679724,
85.2338219878376));
#179146=CARTESIAN_POINT('Ctrl Pts',(-27.3284384471618,-73.8432844854502,
85.1964254653508));
#179147=CARTESIAN_POINT('Ctrl Pts',(-27.3416352450666,-73.2992036660809,
85.1325800364409));
#179148=CARTESIAN_POINT('Ctrl Pts',(-27.3663355732002,-72.2793557765799,
84.9430020041002));
#179149=CARTESIAN_POINT('Ctrl Pts',(-27.3778535281864,-71.803301281166,
84.8245912456166));
#179150=CARTESIAN_POINT('Ctrl Pts',(-27.4049057657027,-70.6883464213871,
84.4750671390777));
#179151=CARTESIAN_POINT('Ctrl Pts',(-27.4202067577981,-70.0590493170962,
84.2187440789919));
#179152=CARTESIAN_POINT('Ctrl Pts',(-27.4436576488854,-69.1493981606462,
83.7568893364926));
#179153=CARTESIAN_POINT('Ctrl Pts',(-27.4516265373343,-68.8511998500405,
83.5894374249849));
#179154=CARTESIAN_POINT('Ctrl Pts',(-27.4724757847193,-68.1038032722249,
83.1275803988205));
#179155=CARTESIAN_POINT('Ctrl Pts',(-27.4854181878823,-67.6662498040756,
82.8157248435304));
#179156=CARTESIAN_POINT('Ctrl Pts',(-27.5104501434681,-66.8526039734047,
82.1511201466782));
#179157=CARTESIAN_POINT('Ctrl Pts',(-27.5225285306441,-66.4754907525204,
81.8013399821767));
#179158=CARTESIAN_POINT('Ctrl Pts',(-27.5502539247456,-65.6500072137001,
80.9329664608923));
#179159=CARTESIAN_POINT('Ctrl Pts',(-27.5656791229289,-65.2209437995513,
80.3983953344034));
#179160=CARTESIAN_POINT('Ctrl Pts',(-27.5957935746758,-64.4899240356691,
79.3127252958504));
#179161=CARTESIAN_POINT('Ctrl Pts',(-27.6106797998656,-64.1812230031144,
78.7687359234635));
#179162=CARTESIAN_POINT('Ctrl Pts',(-27.6444527628368,-63.5811713203051,
77.4932371811879));
#179163=CARTESIAN_POINT('Ctrl Pts',(-27.6630708869892,-63.316038462461,
76.7523815074266));
#179164=CARTESIAN_POINT('Ctrl Pts',(-27.6975854290323,-62.9498407995109,
75.3038255052403));
#179165=CARTESIAN_POINT('Ctrl Pts',(-27.7135322676883,-62.8360710496892,
74.6026073933139));
#179166=CARTESIAN_POINT('Ctrl Pts',(-27.7412936953252,-62.7471464229716,
73.404366222219));
#179167=CARTESIAN_POINT('Ctrl Pts',(-27.7530105228034,-62.7403494745055,
72.9114909306455));
#179168=CARTESIAN_POINT('Ctrl Pts',(-27.7757173040353,-62.784414674497,
71.9643874888223));
#179169=CARTESIAN_POINT('Ctrl Pts',(-27.7866415926275,-62.8309722130037,
71.5107501260004));
#179170=CARTESIAN_POINT('Ctrl Pts',(-27.8157863163464,-63.024804177098,
70.2946245194572));
#179171=CARTESIAN_POINT('Ctrl Pts',(-27.8335928030878,-63.2194193437323,
69.5418161954899));
#179172=CARTESIAN_POINT('Ctrl Pts',(-27.8653577822833,-63.6940768218159,
68.2329906182506));
#179173=CARTESIAN_POINT('Ctrl Pts',(-27.8794342347984,-63.9476674362967,
67.6702035356999));
#179174=CARTESIAN_POINT('Ctrl Pts',(-27.9071511898918,-64.5061430050634,
66.6449859021958));
#179175=CARTESIAN_POINT('Ctrl Pts',(-27.9204412958119,-64.8020938015374,
66.1794211021552));
#179176=CARTESIAN_POINT('Ctrl Pts',(-27.9450383556779,-65.4138928553907,
65.3467986623169));
#179177=CARTESIAN_POINT('Ctrl Pts',(-27.9563686515075,-65.7221002081431,
64.9754267364466));
#179178=CARTESIAN_POINT('Ctrl Pts',(-27.9832040188346,-66.5135494043126,
64.128831251076));
#179179=CARTESIAN_POINT('Ctrl Pts',(-27.998471703676,-67.0158708779765,
63.6736250058297));
#179180=CARTESIAN_POINT('Ctrl Pts',(-28.0307468331084,-68.1309914402376,
62.8198807146967));
#179181=CARTESIAN_POINT('Ctrl Pts',(-28.0481682387343,-68.7470322616654,
62.4298951177045));
#179182=CARTESIAN_POINT('Ctrl Pts',(-28.0837083826578,-70.0670980213893,
61.7504714027153));
#179183=CARTESIAN_POINT('Ctrl Pts',(-28.1015536528359,-70.770857774297,
61.4671731473188));
#179184=CARTESIAN_POINT('Ctrl Pts',(-28.1322886314172,-72.0496074031833,
61.085479821206));
#179185=CARTESIAN_POINT('Ctrl Pts',(-28.1453419850708,-72.6139403548083,
60.959646209966));
#179186=CARTESIAN_POINT('Ctrl Pts',(-28.1642049393277,-73.4257058037411,
60.8380326655313));
#179187=CARTESIAN_POINT('Ctrl Pts',(-28.1698402086512,-73.667394819608,
60.8091568487183));
#179188=CARTESIAN_POINT('Ctrl Pts',(-28.1841216233844,-74.2722848219316,
60.7551088154341));
#179189=CARTESIAN_POINT('Ctrl Pts',(-28.1928337586347,-74.6360383204453,
60.738889950456));
#179190=CARTESIAN_POINT('Ctrl Pts',(-28.2015531594526,-74.9999810209095,
60.7388893865947));
#179191=CARTESIAN_POINT('',(-28.5675342178229,-86.7327262929796,69.46672519));
#179192=CARTESIAN_POINT('Ctrl Pts',(-28.2015531594526,-74.9999810209094,
60.7388893865947));
#179193=CARTESIAN_POINT('Ctrl Pts',(-28.2115085777165,-75.4155143680877,
60.7388887428033));
#179194=CARTESIAN_POINT('Ctrl Pts',(-28.2214581486582,-75.8307807951183,
60.7600311204054));
#179195=CARTESIAN_POINT('Ctrl Pts',(-28.2563764973937,-77.2985729646583,
60.9098820884177));
#179196=CARTESIAN_POINT('Ctrl Pts',(-28.2802056089585,-78.3345430940372,
61.1539135737514));
#179197=CARTESIAN_POINT('Ctrl Pts',(-28.3161178277994,-79.7947420362231,
61.7051026614067));
#179198=CARTESIAN_POINT('Ctrl Pts',(-28.3279543485361,-80.2520597013501,
61.9105662236378));
#179199=CARTESIAN_POINT('Ctrl Pts',(-28.3551888069236,-81.2597771872479,
62.4397707987469));
#179200=CARTESIAN_POINT('Ctrl Pts',(-28.3704805414799,-81.8000694228291,
62.7796884624179));
#179201=CARTESIAN_POINT('Ctrl Pts',(-28.4005460677347,-82.8274228573546,
63.543917669771));
#179202=CARTESIAN_POINT('Ctrl Pts',(-28.4152665757593,-83.3123674267628,
63.9677699594752));
#179203=CARTESIAN_POINT('Ctrl Pts',(-28.4443880543649,-84.2043832438057,
64.8806906223373));
#179204=CARTESIAN_POINT('Ctrl Pts',(-28.458867085717,-84.6111720028112,
65.3672798388122));
#179205=CARTESIAN_POINT('Ctrl Pts',(-28.4987753663392,-85.5849460603147,
66.7347398350442));
#179206=CARTESIAN_POINT('Ctrl Pts',(-28.5239637024403,-86.0798870006963,
67.6605065258182));
#179207=CARTESIAN_POINT('Ctrl Pts',(-28.554878072722,-86.5549068914363,
68.9106765416828));
#179208=CARTESIAN_POINT('Ctrl Pts',(-28.5615651320878,-86.648794391744,
69.1871419701532));
#179209=CARTESIAN_POINT('Ctrl Pts',(-28.568231723297,-86.7327175810979,
69.4666971484707));
#179210=CARTESIAN_POINT('Origin',(-28.5675339373409,-75.,72.98888938658));
#179211=CARTESIAN_POINT('Origin',(-23.90845228375,-75.0031087425464,72.9873550812444));
#179212=CARTESIAN_POINT('Ctrl Pts',(-19.9173382169355,-75.0031141882852,
59.938705268027));
#179213=CARTESIAN_POINT('Ctrl Pts',(-19.9328718779449,-75.715458030901,
59.9387055653175));
#179214=CARTESIAN_POINT('Ctrl Pts',(-19.9485771854427,-76.4265935451757,
59.9970363718849));
#179215=CARTESIAN_POINT('Ctrl Pts',(-19.9794959376743,-77.8228375541618,
60.2276392928315));
#179216=CARTESIAN_POINT('Ctrl Pts',(-19.9946414269002,-78.5058787600641,
60.3980014898524));
#179217=CARTESIAN_POINT('Ctrl Pts',(-20.020231467096,-79.6151980199155,
60.7720050886729));
#179218=CARTESIAN_POINT('Ctrl Pts',(-20.0305208112033,-80.0501671806586,
60.9452065047758));
#179219=CARTESIAN_POINT('Ctrl Pts',(-20.054213345243,-81.0286408710152,
61.3971744171832));
#179220=CARTESIAN_POINT('Ctrl Pts',(-20.067452530708,-81.5637737295914,
61.6914708006862));
#179221=CARTESIAN_POINT('Ctrl Pts',(-20.1027340705551,-82.9258791914871,
62.5701115632893));
#179222=CARTESIAN_POINT('Ctrl Pts',(-20.1250778021996,-83.708848783791,
63.2149789388751));
#179223=CARTESIAN_POINT('Ctrl Pts',(-20.1617910749169,-84.8732817561689,
64.4261200658439));
#179224=CARTESIAN_POINT('Ctrl Pts',(-20.1762912027402,-85.2992739037134,
64.9434726307752));
#179225=CARTESIAN_POINT('Ctrl Pts',(-20.2096346355115,-86.1717387900149,
66.1865703941092));
#179226=CARTESIAN_POINT('Ctrl Pts',(-20.2284294933597,-86.590705502097,
66.9279345931321));
#179227=CARTESIAN_POINT('Ctrl Pts',(-20.2654139263425,-87.2765823618294,
68.4770834263672));
#179228=CARTESIAN_POINT('Ctrl Pts',(-20.2838971286937,-87.5427332229182,
69.2808047207612));
#179229=CARTESIAN_POINT('Ctrl Pts',(-20.3216439621127,-87.9198791768367,
70.9457471846908));
#179230=CARTESIAN_POINT('Ctrl Pts',(-20.3404122468529,-88.0265554601149,
71.8037332445827));
#179231=CARTESIAN_POINT('Ctrl Pts',(-20.3776586003379,-88.0683398576455,
73.4995953867203));
#179232=CARTESIAN_POINT('Ctrl Pts',(-20.3962184666146,-88.0089189581226,
74.3332937421367));
#179233=CARTESIAN_POINT('Ctrl Pts',(-20.4297101871404,-87.7558015577041,
75.8353949195096));
#179234=CARTESIAN_POINT('Ctrl Pts',(-20.4447248012191,-87.5875584191361,
76.5050437589806));
#179235=CARTESIAN_POINT('Ctrl Pts',(-20.4785976203819,-87.0971503765792,
77.9587940353662));
#179236=CARTESIAN_POINT('Ctrl Pts',(-20.4973862173595,-86.7499859099212,
78.7312154115928));
#179237=CARTESIAN_POINT('Ctrl Pts',(-20.5345168439657,-85.9099603117664,
80.2002547050643));
#179238=CARTESIAN_POINT('Ctrl Pts',(-20.5531508569545,-85.4186623477612,
80.8931484026368));
#179239=CARTESIAN_POINT('Ctrl Pts',(-20.5911521673481,-84.2980486921671,
82.1861153972118));
#179240=CARTESIAN_POINT('Ctrl Pts',(-20.6100199719696,-83.6690299106182,
82.7809710848248));
#179241=CARTESIAN_POINT('Ctrl Pts',(-20.6480352022366,-82.3046339052498,
83.8361641127842));
#179242=CARTESIAN_POINT('Ctrl Pts',(-20.6672699340158,-81.5729076168941,
84.2942852396785));
#179243=CARTESIAN_POINT('Ctrl Pts',(-20.6954072800321,-80.4284917150397,
84.8619396704294));
#179244=CARTESIAN_POINT('Ctrl Pts',(-20.7045221586876,-80.0469423802783,
85.0289613853488));
#179245=CARTESIAN_POINT('Ctrl Pts',(-20.731735648922,-78.8918403432668,
85.470052613439));
#179246=CARTESIAN_POINT('Ctrl Pts',(-20.7500010159105,-78.0997385821004,
85.6897502466688));
#179247=CARTESIAN_POINT('Ctrl Pts',(-20.7839394540462,-76.5895390569253,
85.9588632142663));
#179248=CARTESIAN_POINT('Ctrl Pts',(-20.7994854167175,-75.8777092140418,
86.0262147262174));
#179249=CARTESIAN_POINT('Ctrl Pts',(-20.8298991951288,-74.5003608331042,
86.0431939440437));
#179250=CARTESIAN_POINT('Ctrl Pts',(-20.8446904689427,-73.8371128676917,
86.0007379283836));
#179251=CARTESIAN_POINT('Ctrl Pts',(-20.8685712035894,-72.7666536364926,
85.8496943995477));
#179252=CARTESIAN_POINT('Ctrl Pts',(-20.8777014719356,-72.3563606926527,
85.7715730814768));
#179253=CARTESIAN_POINT('Ctrl Pts',(-20.9065548531477,-71.0782696750546,
85.4640440639101));
#179254=CARTESIAN_POINT('Ctrl Pts',(-20.9264586059087,-70.2299859384139,
85.1647691514107));
#179255=CARTESIAN_POINT('Ctrl Pts',(-20.9624085347492,-68.7596563066096,
84.468600318769));
#179256=CARTESIAN_POINT('Ctrl Pts',(-20.9782587817702,-68.1275196936063,
84.1015787332102));
#179257=CARTESIAN_POINT('Ctrl Pts',(-21.0071336160251,-67.0526430909996,
83.3505400372593));
#179258=CARTESIAN_POINT('Ctrl Pts',(-21.0200370278404,-66.5987049877021,
82.9859300348966));
#179259=CARTESIAN_POINT('Ctrl Pts',(-21.0492239418947,-65.6262671838517,
82.0916936008069));
#179260=CARTESIAN_POINT('Ctrl Pts',(-21.0652641583058,-65.1254637681109,
81.5457584363112));
#179261=CARTESIAN_POINT('Ctrl Pts',(-21.0948863457614,-64.3013963644586,
80.4781289460507));
#179262=CARTESIAN_POINT('Ctrl Pts',(-21.1083724510535,-63.9634103086122,
79.9704343269327));
#179263=CARTESIAN_POINT('Ctrl Pts',(-21.1381836626386,-63.2949339790157,
78.7957212388062));
#179264=CARTESIAN_POINT('Ctrl Pts',(-21.1542576021094,-62.9834791987738,
78.1202860235758));
#179265=CARTESIAN_POINT('Ctrl Pts',(-21.1860047343489,-62.4912225679133,
76.7580814372926));
#179266=CARTESIAN_POINT('Ctrl Pts',(-21.2016346300804,-62.3055693523857,
76.0757463349101));
#179267=CARTESIAN_POINT('Ctrl Pts',(-21.2333295592881,-62.0405658640461,
74.6560915237694));
#179268=CARTESIAN_POINT('Ctrl Pts',(-21.2492757946066,-61.9669310189405,
73.9202395860471));
#179269=CARTESIAN_POINT('Ctrl Pts',(-21.2746493609849,-61.9496509779779,
72.7626619893793));
#179270=CARTESIAN_POINT('Ctrl Pts',(-21.2838878379608,-61.963621017613,
72.3431459475744));
#179271=CARTESIAN_POINT('Ctrl Pts',(-21.3121226657287,-62.0680418283112,
71.0647864277703));
#179272=CARTESIAN_POINT('Ctrl Pts',(-21.3307504508386,-62.2234892052623,
70.2136295091217));
#179273=CARTESIAN_POINT('Ctrl Pts',(-21.3655718339773,-62.663661937125,
68.6816007166605));
#179274=CARTESIAN_POINT('Ctrl Pts',(-21.3817119942731,-62.9241567238436,
67.9973268503584));
#179275=CARTESIAN_POINT('Ctrl Pts',(-21.4142593504455,-63.5693474987497,
66.6538600285569));
#179276=CARTESIAN_POINT('Ctrl Pts',(-21.4306247728224,-63.9572718921026,
65.9992544828227));
#179277=CARTESIAN_POINT('Ctrl Pts',(-21.4583442250649,-64.6956589934538,
64.9697989149321));
#179278=CARTESIAN_POINT('Ctrl Pts',(-21.4695135597142,-65.0151944244029,
64.5750846690903));
#179279=CARTESIAN_POINT('Ctrl Pts',(-21.4994709654415,-65.9366671084101,
63.5635515538473));
#179280=CARTESIAN_POINT('Ctrl Pts',(-21.5179575508267,-66.577997966108,
62.9860578253547));
#179281=CARTESIAN_POINT('Ctrl Pts',(-21.5458585159931,-67.60573646322,62.2301116846202));
#179282=CARTESIAN_POINT('Ctrl Pts',(-21.5549743395996,-67.9514941991276,
62.0003566892381));
#179283=CARTESIAN_POINT('Ctrl Pts',(-21.5829649984971,-69.0472703839904,
61.3452814151252));
#179284=CARTESIAN_POINT('Ctrl Pts',(-21.6014757670978,-69.8289194391713,
60.9774568428056));
#179285=CARTESIAN_POINT('Ctrl Pts',(-21.6348096952452,-71.2682548922788,
60.4669345020941));
#179286=CARTESIAN_POINT('Ctrl Pts',(-21.6494761519027,-71.9115034436083,
60.2927878034823));
#179287=CARTESIAN_POINT('Ctrl Pts',(-21.6730783604569,-72.9745208716184,
60.0906236826485));
#179288=CARTESIAN_POINT('Ctrl Pts',(-21.6820869004331,-73.3873171477512,
60.0324306001988));
#179289=CARTESIAN_POINT('Ctrl Pts',(-21.6998459227287,-74.2016867105178,
59.957161428136));
#179290=CARTESIAN_POINT('Ctrl Pts',(-21.7085784447897,-74.6024198115221,
59.9387052680259));
#179291=CARTESIAN_POINT('Ctrl Pts',(-21.7173525905574,-75.0031087425464,
59.9387052680259));
#179292=CARTESIAN_POINT('Ctrl Pts',(-21.4178560137238,-75.0031087349823,
59.9387052680259));
#179293=CARTESIAN_POINT('Ctrl Pts',(-21.4165790214011,-74.9450765584729,
59.9387052680596));
#179294=CARTESIAN_POINT('Ctrl Pts',(-21.4153012122267,-74.8870410412435,
59.9390924039174));
#179295=CARTESIAN_POINT('Ctrl Pts',(-21.3982849488851,-74.114761740527,
59.9493975218163));
#179296=CARTESIAN_POINT('Ctrl Pts',(-21.3823795244862,-73.4025083610337,
60.0175605981627));
#179297=CARTESIAN_POINT('Ctrl Pts',(-21.3479674952683,-71.8722695165063,
60.2920289451095));
#179298=CARTESIAN_POINT('Ctrl Pts',(-21.3296902599154,-71.0613777063911,
60.519948827425));
#179299=CARTESIAN_POINT('Ctrl Pts',(-21.2919933924485,-69.4744729716801,
61.136421088153));
#179300=CARTESIAN_POINT('Ctrl Pts',(-21.2728381923279,-68.7038021304673,
61.5274600692303));
#179301=CARTESIAN_POINT('Ctrl Pts',(-21.2354813627788,-67.2705110473185,
62.4432674643334));
#179302=CARTESIAN_POINT('Ctrl Pts',(-21.2169686074118,-66.6088707468293,
62.9620066918454));
#179303=CARTESIAN_POINT('Ctrl Pts',(-21.1793329586012,-65.3823273712759,
64.1307437952212));
#179304=CARTESIAN_POINT('Ctrl Pts',(-21.1606856991897,-64.8225650507218,
64.7803135541843));
#179305=CARTESIAN_POINT('Ctrl Pts',(-21.1257642338435,-63.9114446212539,
66.0755869885543));
#179306=CARTESIAN_POINT('Ctrl Pts',(-21.1095322663368,-63.5430737896763,
66.7052261979723));
#179307=CARTESIAN_POINT('Ctrl Pts',(-21.0779527528966,-62.9262938930541,
67.9962232652629));
#179308=CARTESIAN_POINT('Ctrl Pts',(-21.0626602223071,-62.6751226930866,
68.6535785836184));
#179309=CARTESIAN_POINT('Ctrl Pts',(-21.0281203676375,-62.236057338798,
70.1563637592512));
#179310=CARTESIAN_POINT('Ctrl Pts',(-21.0089201382509,-62.0768047623284,
71.006752535638));
#179311=CARTESIAN_POINT('Ctrl Pts',(-20.9808474681184,-61.9667648876738,
72.2832005045049));
#179312=CARTESIAN_POINT('Ctrl Pts',(-20.9717060177443,-61.9508962789211,
72.7012706524723));
#179313=CARTESIAN_POINT('Ctrl Pts',(-20.9460321822843,-61.9627084972529,
73.8686767451884));
#179314=CARTESIAN_POINT('Ctrl Pts',(-20.9293704136499,-62.0348199990523,
74.6159276773357));
#179315=CARTESIAN_POINT('Ctrl Pts',(-20.8989581724167,-62.2855868778281,
75.9763025640758));
#179316=CARTESIAN_POINT('Ctrl Pts',(-20.8851892419988,-62.4457958755654,
76.590557376275));
#179317=CARTESIAN_POINT('Ctrl Pts',(-20.8550000675132,-62.8885918857284,
77.8918693461325));
#179318=CARTESIAN_POINT('Ctrl Pts',(-20.8385582738716,-63.1864282792172,
78.5714252713954));
#179319=CARTESIAN_POINT('Ctrl Pts',(-20.8068765314766,-63.8767920825402,
79.8406983324079));
#179320=CARTESIAN_POINT('Ctrl Pts',(-20.7916154146475,-64.2628204105242,
80.4311072859444));
#179321=CARTESIAN_POINT('Ctrl Pts',(-20.7598032915303,-65.1509763675334,
81.5755355948962));
#179322=CARTESIAN_POINT('Ctrl Pts',(-20.7433179736035,-65.6568374527347,
82.1234689105735));
#179323=CARTESIAN_POINT('Ctrl Pts',(-20.7130362566075,-66.6818828118141,
83.0590204971938));
#179324=CARTESIAN_POINT('Ctrl Pts',(-20.6990820858438,-67.1885491305867,
83.4570209699789));
#179325=CARTESIAN_POINT('Ctrl Pts',(-20.6683120568835,-68.3527778080183,
84.2397853814381));
#179326=CARTESIAN_POINT('Ctrl Pts',(-20.651540366393,-69.018853690199,84.6077160095614));
#179327=CARTESIAN_POINT('Ctrl Pts',(-20.6259743233929,-70.0928167066275,
85.0839993296045));
#179328=CARTESIAN_POINT('Ctrl Pts',(-20.6169658493251,-70.4803181726352,
85.2341561079651));
#179329=CARTESIAN_POINT('Ctrl Pts',(-20.5890207711908,-71.6956057981309,
85.639518631415));
#179330=CARTESIAN_POINT('Ctrl Pts',(-20.5698924184271,-72.5421199886465,
85.8310443509021));
#179331=CARTESIAN_POINT('Ctrl Pts',(-20.539134914783,-73.9442761892445,
86.0044754413283));
#179332=CARTESIAN_POINT('Ctrl Pts',(-20.5273091091971,-74.4908961418339,
86.0374197567479));
#179333=CARTESIAN_POINT('Ctrl Pts',(-20.4995210326799,-75.7648514863862,
86.0340165646542));
#179334=CARTESIAN_POINT('Ctrl Pts',(-20.4834920933317,-76.4903019509806,
85.9713405663449));
#179335=CARTESIAN_POINT('Ctrl Pts',(-20.4535479370001,-77.8431237815135,
85.7395487093813));
#179336=CARTESIAN_POINT('Ctrl Pts',(-20.4396368488468,-78.4705327621653,
85.5834299595451));
#179337=CARTESIAN_POINT('Ctrl Pts',(-20.4101052979605,-79.7569333901446,
85.1598911830048));
#179338=CARTESIAN_POINT('Ctrl Pts',(-20.3944867931946,-80.4108891481077,
84.8837995041944));
#179339=CARTESIAN_POINT('Ctrl Pts',(-20.3649983002911,-81.6094682018597,
84.2584261003021));
#179340=CARTESIAN_POINT('Ctrl Pts',(-20.3511423230588,-82.1569732220308,
83.9191094746264));
#179341=CARTESIAN_POINT('Ctrl Pts',(-20.3219006509759,-83.2417719994142,
83.1302807342162));
#179342=CARTESIAN_POINT('Ctrl Pts',(-20.306521295237,-83.7724726487,82.6751186986466));
#179343=CARTESIAN_POINT('Ctrl Pts',(-20.2767885721029,-84.7317940630188,
81.7086218141905));
#179344=CARTESIAN_POINT('Ctrl Pts',(-20.2624929320801,-85.1627526688423,
81.2025513754549));
#179345=CARTESIAN_POINT('Ctrl Pts',(-20.2330980141271,-85.9556603416621,
80.1131055038267));
#179346=CARTESIAN_POINT('Ctrl Pts',(-20.2180277182533,-86.31391656035,79.5295509346996));
#179347=CARTESIAN_POINT('Ctrl Pts',(-20.1867522576109,-86.9644172258488,
78.2553940587279));
#179348=CARTESIAN_POINT('Ctrl Pts',(-20.1706664885413,-87.2462963892034,
77.5622315936384));
#179349=CARTESIAN_POINT('Ctrl Pts',(-20.139673070264,-87.6655309470806,
76.208990273409));
#179350=CARTESIAN_POINT('Ctrl Pts',(-20.1248759571721,-87.8141821205888,
75.5548963316572));
#179351=CARTESIAN_POINT('Ctrl Pts',(-20.0917409474285,-88.0356832969413,
74.0538869219616));
#179352=CARTESIAN_POINT('Ctrl Pts',(-20.07343120113,-88.0774324955213,73.2054210066669));
#179353=CARTESIAN_POINT('Ctrl Pts',(-20.0456647480087,-88.0166106702952,
71.9440021368037));
#179354=CARTESIAN_POINT('Ctrl Pts',(-20.0364949274527,-87.9768030491948,
71.5302780244807));
#179355=CARTESIAN_POINT('Ctrl Pts',(-20.0084293209196,-87.7938052083768,
70.265274237822));
#179356=CARTESIAN_POINT('Ctrl Pts',(-19.9898157937922,-87.5858969951755,
69.4257428314119));
#179357=CARTESIAN_POINT('Ctrl Pts',(-19.9518799915304,-87.0076193181874,
67.8006083720809));
#179358=CARTESIAN_POINT('Ctrl Pts',(-19.9328676430594,-86.6387824155251,
67.0189616610644));
#179359=CARTESIAN_POINT('Ctrl Pts',(-19.9047804306668,-85.9773877236089,
65.9153979274948));
#179360=CARTESIAN_POINT('Ctrl Pts',(-19.8955052982431,-85.7415868499336,
65.562231245798));
#179361=CARTESIAN_POINT('Ctrl Pts',(-19.8716429626955,-85.0960133134504,
64.6905773924108));
#179362=CARTESIAN_POINT('Ctrl Pts',(-19.8569765233847,-84.663321493607,
64.1905640763602));
#179363=CARTESIAN_POINT('Ctrl Pts',(-19.8240096264381,-83.5979057628111,
63.1332419920548));
#179364=CARTESIAN_POINT('Ctrl Pts',(-19.8057428004871,-82.9453214349789,
62.6000867805438));
#179365=CARTESIAN_POINT('Ctrl Pts',(-19.7733639122021,-81.7270753051805,
61.7871439521476));
#179366=CARTESIAN_POINT('Ctrl Pts',(-19.759512466268,-81.183982720971,61.4785211743792));
#179367=CARTESIAN_POINT('Ctrl Pts',(-19.7353152738702,-80.1884174905541,
61.003639661926));
#179368=CARTESIAN_POINT('Ctrl Pts',(-19.7248456932155,-79.7448982524453,
60.8213247415312));
#179369=CARTESIAN_POINT('Ctrl Pts',(-19.6983318520157,-78.6076162272353,
60.4254897365281));
#179370=CARTESIAN_POINT('Ctrl Pts',(-19.6821871197268,-77.9042029224063,
60.2446481322081));
#179371=CARTESIAN_POINT('Ctrl Pts',(-19.650007434917,-76.4671189013943,
60.0004104549331));
#179372=CARTESIAN_POINT('Ctrl Pts',(-19.6340602481707,-75.7357661204461,
59.9387048126255));
#179373=CARTESIAN_POINT('Ctrl Pts',(-19.6178714446467,-75.0031006318965,
59.9387052680284));
#179374=CARTESIAN_POINT('Origin',(-29.0675369414309,-75.,72.98888938658));
#179375=CARTESIAN_POINT('',(-29.3659074908668,-88.048139596166,72.910724257937));
#179376=CARTESIAN_POINT('',(-29.0715747727696,-75.,60.2348484464093));
#179377=CARTESIAN_POINT('Ctrl Pts',(-29.3659074908668,-88.048139596166,
72.910724257937));
#179378=CARTESIAN_POINT('Ctrl Pts',(-29.3546070927136,-88.0320891389882,
72.1178290339509));
#179379=CARTESIAN_POINT('Ctrl Pts',(-29.3435513987386,-87.943946214938,
71.327216757012));
#179380=CARTESIAN_POINT('Ctrl Pts',(-29.3198744527459,-87.6154974982477,
69.7320276466834));
#179381=CARTESIAN_POINT('Ctrl Pts',(-29.307347194069,-87.3681853141254,
68.9317585165297));
#179382=CARTESIAN_POINT('Ctrl Pts',(-29.2716009614049,-86.4261070896003,
66.6770808862898));
#179383=CARTESIAN_POINT('Ctrl Pts',(-29.2493251734954,-85.5346342704723,
65.3168568070417));
#179384=CARTESIAN_POINT('Ctrl Pts',(-29.2008834203201,-83.2740044679819,
62.978809133931));
#179385=CARTESIAN_POINT('Ctrl Pts',(-29.1779340274024,-81.9179021187915,
62.0244452183611));
#179386=CARTESIAN_POINT('Ctrl Pts',(-29.1412176792203,-79.6470774108627,
61.0067126403781));
#179387=CARTESIAN_POINT('Ctrl Pts',(-29.1283139882113,-78.8387324105875,
60.7373079795366));
#179388=CARTESIAN_POINT('Ctrl Pts',(-29.1035475953469,-77.2063592530559,
60.3677278885152));
#179389=CARTESIAN_POINT('Ctrl Pts',(-29.0916996520762,-76.3859047406108,
60.2633970793085));
#179390=CARTESIAN_POINT('Ctrl Pts',(-29.0770376134035,-75.3744456229184,
60.233503939114));
#179391=CARTESIAN_POINT('Ctrl Pts',(-29.0743156629404,-75.1871357568877,
60.2321075556738));
#179392=CARTESIAN_POINT('Ctrl Pts',(-29.0715747727696,-75.,60.2348484464093));
#179393=CARTESIAN_POINT('',(-29.5675339851921,-75.,59.7388891318012));
#179394=CARTESIAN_POINT('',(-29.0675369414309,-75.,60.23888627858));
#179395=CARTESIAN_POINT('Origin',(-29.5675339847409,-75.,72.98888938658));
#179396=CARTESIAN_POINT('Ctrl Pts',(-29.0715747727696,-75.,60.2348484464093));
#179397=CARTESIAN_POINT('Ctrl Pts',(-29.0624830013418,-74.3792543948848,
60.2439402197103));
#179398=CARTESIAN_POINT('Ctrl Pts',(-29.0530879239002,-73.7604267662681,
60.298613478141));
#179399=CARTESIAN_POINT('Ctrl Pts',(-29.0196088358811,-71.5708262745697,
60.6545856066194));
#179400=CARTESIAN_POINT('Ctrl Pts',(-28.9970544073908,-70.0494382406995,
61.2063873466819));
#179401=CARTESIAN_POINT('Ctrl Pts',(-28.9605640939231,-67.9680269694554,
62.4497133389986));
#179402=CARTESIAN_POINT('Ctrl Pts',(-28.9479315721134,-67.3041712311103,
62.9401165236319));
#179403=CARTESIAN_POINT('Ctrl Pts',(-28.9236753448913,-66.0997830229611,
64.0256989173661));
#179404=CARTESIAN_POINT('Ctrl Pts',(-28.9120635621393,-65.5579519187452,
64.6158534956667));
#179405=CARTESIAN_POINT('Ctrl Pts',(-28.8757570605804,-64.0709138031728,
66.5825031309042));
#179406=CARTESIAN_POINT('Ctrl Pts',(-28.8499124305472,-63.3442409609021,
68.094175332673));
#179407=CARTESIAN_POINT('Ctrl Pts',(-28.8133913070736,-62.7300938236352,
70.4880258732612));
#179408=CARTESIAN_POINT('Ctrl Pts',(-28.8014073382016,-62.6053405970239,
71.2917639575562));
#179409=CARTESIAN_POINT('Ctrl Pts',(-28.7766246431217,-62.5156428752478,
72.9010220163151));
#179410=CARTESIAN_POINT('Ctrl Pts',(-28.7642803679076,-62.5480378309257,
73.7016986295373));
#179411=CARTESIAN_POINT('Ctrl Pts',(-28.7402659878244,-62.7645775607116,
75.2800816269133));
#179412=CARTESIAN_POINT('Ctrl Pts',(-28.7286237203234,-62.9475553373186,
76.0555728904185));
#179413=CARTESIAN_POINT('Ctrl Pts',(-28.6920185593442,-63.730299249319,
78.3547530244634));
#179414=CARTESIAN_POINT('Ctrl Pts',(-28.6664353682654,-64.5592604210176,
79.7818999885085));
#179415=CARTESIAN_POINT('Ctrl Pts',(-28.6175016536543,-66.7203052977945,
82.2305946258992));
#179416=CARTESIAN_POINT('Ctrl Pts',(-28.5917552851516,-68.0293736273903,
83.2219482748759));
#179417=CARTESIAN_POINT('Ctrl Pts',(-28.5670511147326,-69.4942820408445,
83.9313635516326));
#179418=CARTESIAN_POINT('',(-29.3655838523951,-81.601362674698,84.2438270474906));
#179419=CARTESIAN_POINT('Ctrl Pts',(-29.3655838526627,-81.6013626745626,
84.2438270472598));
#179420=CARTESIAN_POINT('Ctrl Pts',(-29.3515369276678,-81.860548904277,
84.075521599617));
#179421=CARTESIAN_POINT('Ctrl Pts',(-29.3375494753961,-82.1133189850824,
83.8983413632426));
#179422=CARTESIAN_POINT('Ctrl Pts',(-29.3235615282547,-82.3590602344623,
83.7127408512463));
#179423=CARTESIAN_POINT('Ctrl Pts',(-29.309689642279,-82.6027625130371,
83.5286803087355));
#179424=CARTESIAN_POINT('Ctrl Pts',(-29.2958172696116,-82.8395518899398,
83.3363387224601));
#179425=CARTESIAN_POINT('Ctrl Pts',(-29.281885923003,-83.0688548794704,
83.1362046562238));
#179426=CARTESIAN_POINT('Ctrl Pts',(-29.276907265287,-83.1508010925813,
83.064682567148));
#179427=CARTESIAN_POINT('Ctrl Pts',(-29.271921075776,-83.2317914308853,
82.9921656866292));
#179428=CARTESIAN_POINT('Ctrl Pts',(-29.2669246850387,-83.3118005600568,
82.9186776996054));
#179429=CARTESIAN_POINT('Ctrl Pts',(-29.253192592924,-83.5316978398292,
82.7167031423289));
#179430=CARTESIAN_POINT('Ctrl Pts',(-29.2393423955424,-83.7441786587935,
82.5073393284883));
#179431=CARTESIAN_POINT('Ctrl Pts',(-29.2254372276084,-83.9488227354,82.2911763378452));
#179432=CARTESIAN_POINT('Ctrl Pts',(-29.2113899558856,-84.155558171046,
82.0728042706827));
#179433=CARTESIAN_POINT('Ctrl Pts',(-29.1972865843269,-84.3542958316679,
81.8474936242021));
#179434=CARTESIAN_POINT('Ctrl Pts',(-29.1831922031099,-84.5446534894828,
81.6158677489123));
#179435=CARTESIAN_POINT('Ctrl Pts',(-29.1776338924619,-84.6197236170793,
81.5245229392932));
#179436=CARTESIAN_POINT('Ctrl Pts',(-29.1720769800155,-84.693491022277,
81.4321961088974));
#179437=CARTESIAN_POINT('Ctrl Pts',(-29.1665254579116,-84.7659344267727,
81.3389259770428));
#179438=CARTESIAN_POINT('Ctrl Pts',(-29.1526002959194,-84.947647860313,
81.1049718162184));
#179439=CARTESIAN_POINT('Ctrl Pts',(-29.1387540387589,-85.1210444797053,
80.8651301507358));
#179440=CARTESIAN_POINT('Ctrl Pts',(-29.1249636357172,-85.2857375273847,
80.6200008365142));
#179441=CARTESIAN_POINT('Ctrl Pts',(-29.1112138923695,-85.4499449932503,
80.3755942628011));
#179442=CARTESIAN_POINT('Ctrl Pts',(-29.097519674265,-85.6054999816377,
80.1259313935929));
#179443=CARTESIAN_POINT('Ctrl Pts',(-29.0838581339785,-85.7520621961525,
79.871635550916));
#179444=CARTESIAN_POINT('Ctrl Pts',(-29.0702192763375,-85.8983810692383,
79.6177619228867));
#179445=CARTESIAN_POINT('Ctrl Pts',(-29.0566129880928,-86.0357368606978,
79.3592709194749));
#179446=CARTESIAN_POINT('Ctrl Pts',(-29.0430165354333,-86.1638361835182,
79.0968081432393));
#179447=CARTESIAN_POINT('Ctrl Pts',(-29.0294524529149,-86.2916305302353,
78.8349702327174));
#179448=CARTESIAN_POINT('Ctrl Pts',(-29.0158981592047,-86.4102123109604,
78.5691796794727));
#179449=CARTESIAN_POINT('Ctrl Pts',(-29.0023310824778,-86.5193372434198,
78.300099265784));
#179450=CARTESIAN_POINT('Ctrl Pts',(-28.990922018484,-86.6111044945981,
78.0738194472896));
#179451=CARTESIAN_POINT('Ctrl Pts',(-28.9795039146485,-86.6961848660042,
77.8452135701712));
#179452=CARTESIAN_POINT('Ctrl Pts',(-28.968063347715,-86.7744598057493,
77.6146858321683));
#179453=CARTESIAN_POINT('Ctrl Pts',(-28.9545124222423,-86.8671735568285,
77.3416343116225));
#179454=CARTESIAN_POINT('Ctrl Pts',(-28.940872966952,-86.9503156261371,
77.0657889256945));
#179455=CARTESIAN_POINT('Ctrl Pts',(-28.9271816883291,-87.0237753974248,
76.7878423327904));
#179456=CARTESIAN_POINT('Ctrl Pts',(-28.9133962221623,-87.0977405265845,
76.5079836389328));
#179457=CARTESIAN_POINT('Ctrl Pts',(-28.8995582171853,-87.1618897070212,
76.2259950093752));
#179458=CARTESIAN_POINT('Ctrl Pts',(-28.8857051426604,-87.2161629265552,
75.9425807157966));
#179459=CARTESIAN_POINT('Ctrl Pts',(-28.8717987806009,-87.2706449146236,
75.658076234697));
#179460=CARTESIAN_POINT('Ctrl Pts',(-28.8578772328367,-87.3151748930747,
75.3721353741036));
#179461=CARTESIAN_POINT('Ctrl Pts',(-28.8439784026859,-87.3497444916918,
75.0854635881238));
#179462=CARTESIAN_POINT('Ctrl Pts',(-28.8299871301317,-87.3845440159028,
74.7968851216131));
#179463=CARTESIAN_POINT('Ctrl Pts',(-28.8160188783897,-87.4092503014884,
74.5075662463216));
#179464=CARTESIAN_POINT('Ctrl Pts',(-28.8021123121144,-87.4239066307403,
74.2182154033722));
#179465=CARTESIAN_POINT('Ctrl Pts',(-28.7906519385059,-87.4359848825266,
73.9797619491923));
#179466=CARTESIAN_POINT('Ctrl Pts',(-28.7792334578131,-87.4412388178587,
73.7412866412701));
#179467=CARTESIAN_POINT('Ctrl Pts',(-28.7678785097109,-87.4397181565358,
73.5031784169355));
#179468=CARTESIAN_POINT('Ctrl Pts',(-28.7538051587481,-87.4378334451043,
73.2080664905729));
#179469=CARTESIAN_POINT('Ctrl Pts',(-28.7397945616724,-87.425504114295,
72.913559041569));
#179470=CARTESIAN_POINT('Ctrl Pts',(-28.7257924240597,-87.4027855288179,
72.6203915837634));
#179471=CARTESIAN_POINT('Ctrl Pts',(-28.711890316212,-87.3802292424719,
72.3293184827444));
#179472=CARTESIAN_POINT('Ctrl Pts',(-28.6979965473919,-87.3474315684259,
72.0395665459303));
#179473=CARTESIAN_POINT('Ctrl Pts',(-28.6840579785028,-87.3044980173107,
71.7518582558201));
#179474=CARTESIAN_POINT('Ctrl Pts',(-28.679117116274,-87.2892791836744,
71.6498731069271));
#179475=CARTESIAN_POINT('Ctrl Pts',(-28.6741706248307,-87.2727872330889,
71.548144752287));
#179476=CARTESIAN_POINT('Ctrl Pts',(-28.6692161373386,-87.2550284427559,
71.4467053584759));
#179477=CARTESIAN_POINT('Ctrl Pts',(-28.6547265382072,-87.2030921418986,
71.1500417469918));
#179478=CARTESIAN_POINT('Ctrl Pts',(-28.6401112616259,-87.1402582756939,
70.8558425314034));
#179479=CARTESIAN_POINT('Ctrl Pts',(-28.6253112490708,-87.0667134280796,
70.5648824322376));
#179480=CARTESIAN_POINT('Ctrl Pts',(-28.6106590834898,-86.9939032678951,
70.2768289231913));
#179481=CARTESIAN_POINT('Ctrl Pts',(-28.5958258543958,-86.9105950271706,
69.9919503385699));
#179482=CARTESIAN_POINT('Ctrl Pts',(-28.5807542555651,-86.8170207690931,
69.7109948176848));
#179483=CARTESIAN_POINT('Ctrl Pts',(-28.576368234195,-86.789789504499,69.6292332917525));
#179484=CARTESIAN_POINT('Ctrl Pts',(-28.5719620257242,-86.7616891633537,
69.5478039687303));
#179485=CARTESIAN_POINT('Ctrl Pts',(-28.5675342178229,-86.7327262929796,
69.46672519));
#179486=CARTESIAN_POINT('',(-29.3666998404582,-88.0486437994879,72.9886184577035));
#179487=CARTESIAN_POINT('Ctrl Pts',(-29.3655838529309,-81.601362674698,
84.2438270474913));
#179488=CARTESIAN_POINT('Ctrl Pts',(-29.3663355387957,-82.5565513191003,
83.6844513479272));
#179489=CARTESIAN_POINT('Ctrl Pts',(-29.3681108351944,-83.4405607955859,
83.0049447002618));
#179490=CARTESIAN_POINT('Ctrl Pts',(-29.3658391655718,-85.0431672706073,
81.3984887424379));
#179491=CARTESIAN_POINT('Ctrl Pts',(-29.3646108212369,-85.7485241671463,
80.473804649592));
#179492=CARTESIAN_POINT('Ctrl Pts',(-29.3665216258898,-86.8761958843376,
78.5089048792641));
#179493=CARTESIAN_POINT('Ctrl Pts',(-29.3680011405059,-87.3057468920773,
77.4766733383828));
#179494=CARTESIAN_POINT('Ctrl Pts',(-29.3656365873995,-87.8956308654324,
75.2854002296071));
#179495=CARTESIAN_POINT('Ctrl Pts',(-29.3647732455976,-88.0472622045665,
74.1368535505306));
#179496=CARTESIAN_POINT('Ctrl Pts',(-29.3658340844142,-88.0483003098859,
72.9886310426174));
#179497=CARTESIAN_POINT('Ctrl Pts',(-29.3673261860752,-88.0488923027565,
72.9886093529381));
#179498=CARTESIAN_POINT('Ctrl Pts',(-29.3668532876724,-88.0487182780952,
72.9626462799095));
#179499=CARTESIAN_POINT('Ctrl Pts',(-29.3663803892696,-88.0484673808042,
72.9366844270783));
#179500=CARTESIAN_POINT('Ctrl Pts',(-29.3659074908668,-88.048139596166,
72.910724257937));
#179501=CARTESIAN_POINT('Origin',(-28.5675364832709,-75.,72.98888938658));
#179502=CARTESIAN_POINT('',(-27.5675364826718,-60.4999999999999,66.2250147575798));
#179503=CARTESIAN_POINT('',(-27.5675364826401,-60.5,79.7527640156553));
#179504=CARTESIAN_POINT('Ctrl Pts',(-27.5675364817658,-60.5,66.2250147580311));
#179505=CARTESIAN_POINT('Ctrl Pts',(-30.4269114864225,-60.5,72.9888893867033));
#179506=CARTESIAN_POINT('Ctrl Pts',(-27.5675364816388,-60.5,79.7527640154292));
#179507=CARTESIAN_POINT('',(-27.5675364826398,-61.8923127432075,63.8134583462433));
#179508=CARTESIAN_POINT('Origin',(-27.5675364832709,-75.,72.98888938658));
#179509=CARTESIAN_POINT('',(-27.5675364826717,-73.6076872567268,57.0495837172059));
#179510=CARTESIAN_POINT('Ctrl Pts',(-27.5675364817724,-73.6076872563213,
57.0495837174391));
#179511=CARTESIAN_POINT('Ctrl Pts',(-30.4269114864031,-67.7499999999193,
60.4315210317516));
#179512=CARTESIAN_POINT('Ctrl Pts',(-27.5675364816771,-61.8923127434824,
63.8134583460842));
#179513=CARTESIAN_POINT('',(-27.5675364826717,-76.3923127432731,57.0495837172059));
#179514=CARTESIAN_POINT('Origin',(-27.5675364832709,-75.,72.98888938658));
#179515=CARTESIAN_POINT('',(-27.5675364826398,-88.1076872567925,63.8134583462433));
#179516=CARTESIAN_POINT('Ctrl Pts',(-27.567536481677,-88.1076872565176,
63.8134583460842));
#179517=CARTESIAN_POINT('Ctrl Pts',(-30.426911486403,-82.2500000000807,
60.4315210317516));
#179518=CARTESIAN_POINT('Ctrl Pts',(-27.5675364817723,-76.3923127436787,
57.0495837174391));
#179519=CARTESIAN_POINT('',(-27.5675364826718,-89.5000000000001,66.2250147575798));
#179520=CARTESIAN_POINT('Origin',(-27.5675364832709,-75.,72.98888938658));
#179521=CARTESIAN_POINT('',(-27.5675364826718,-89.5,79.7527640155803));
#179522=CARTESIAN_POINT('Ctrl Pts',(-27.5675364817657,-89.5,66.2250147580311));
#179523=CARTESIAN_POINT('Ctrl Pts',(-30.4269114864094,-89.5,72.9888893866725));
#179524=CARTESIAN_POINT('Ctrl Pts',(-27.5675364816705,-89.5,79.7527640153542));
#179525=CARTESIAN_POINT('',(-27.5675364826398,-88.1076872567925,82.1643204269167));
#179526=CARTESIAN_POINT('Origin',(-27.5675364832709,-75.,72.98888938658));
#179527=CARTESIAN_POINT('',(-27.5675364826717,-76.3923127432731,88.9281950559541));
#179528=CARTESIAN_POINT('Ctrl Pts',(-27.5675364817723,-76.3923127436786,
88.9281950557209));
#179529=CARTESIAN_POINT('Ctrl Pts',(-30.426911486403,-82.2500000000806,
85.5462577414084));
#179530=CARTESIAN_POINT('Ctrl Pts',(-27.5675364816771,-88.1076872565176,
82.1643204270758));
#179531=CARTESIAN_POINT('',(-27.5675364816388,-75.,88.9888893864172));
#179532=CARTESIAN_POINT('Origin',(-27.5675364832709,-75.,72.98888938658));
#179533=CARTESIAN_POINT('',(-29.5675364841684,-75.,86.9888893874774));
#179534=CARTESIAN_POINT('',(-28.5675364832709,-75.,87.98888938658));
#179535=CARTESIAN_POINT('Origin',(-29.5675364832709,-75.,72.98888938658));
#179536=CARTESIAN_POINT('',(-27.5675364826399,-73.6076872567918,88.9281950559917));
#179537=CARTESIAN_POINT('Origin',(-27.5675364832709,-75.,72.98888938658));
#179538=CARTESIAN_POINT('',(-27.5675364826716,-61.8923127432725,82.1643204269542));
#179539=CARTESIAN_POINT('Ctrl Pts',(-27.5675364817723,-61.8923127436775,
82.1643204271884));
#179540=CARTESIAN_POINT('Ctrl Pts',(-30.426911486403,-67.7500000000795,
85.5462577415009));
#179541=CARTESIAN_POINT('Ctrl Pts',(-27.5675364816771,-73.6076872565163,
88.9281950558335));
#179542=CARTESIAN_POINT('Origin',(-27.5675364832709,-75.,72.98888938658));
#179543=CARTESIAN_POINT('Origin',(-17.5675364832709,-75.,72.98888938658));
#179544=CARTESIAN_POINT('',(-18.5675364839018,-60.5,66.2250147575047));
#179545=CARTESIAN_POINT('',(-18.56753648387,-60.5,79.7527640155803));
#179546=CARTESIAN_POINT('Ctrl Pts',(-18.5675364848006,-60.5,79.7527640151869));
#179547=CARTESIAN_POINT('Ctrl Pts',(-15.708161480161,-60.5,72.9888893866029));
#179548=CARTESIAN_POINT('Ctrl Pts',(-18.5675364847769,-60.5,66.225014758029));
#179549=CARTESIAN_POINT('',(-18.5675364838598,-61.8923127432938,82.1643204269666));
#179550=CARTESIAN_POINT('Origin',(-18.5675364832709,-75.,72.98888938658));
#179551=CARTESIAN_POINT('',(-18.567536483878,-73.6076872567433,88.9281950559637));
#179552=CARTESIAN_POINT('Ctrl Pts',(-18.5675364847385,-61.8923127437411,
82.1643204272252));
#179553=CARTESIAN_POINT('Ctrl Pts',(-15.7081614801807,-67.7500000000459,
85.5462577414815));
#179554=CARTESIAN_POINT('Ctrl Pts',(-18.5675364847937,-73.6076872563709,
88.9281950557496));
#179555=CARTESIAN_POINT('',(-18.567536483878,-76.3923127432567,88.9281950559637));
#179556=CARTESIAN_POINT('Origin',(-18.5675364832709,-75.,72.98888938658));
#179557=CARTESIAN_POINT('',(-18.5675364838598,-88.1076872567062,82.1643204269666));
#179558=CARTESIAN_POINT('Ctrl Pts',(-18.5675364847937,-76.392312743629,
88.9281950557496));
#179559=CARTESIAN_POINT('Ctrl Pts',(-15.7081614801807,-82.2499999999541,
85.5462577414815));
#179560=CARTESIAN_POINT('Ctrl Pts',(-18.5675364847385,-88.1076872562589,
82.1643204272251));
#179561=CARTESIAN_POINT('',(-18.56753648387,-89.5,79.7527640155802));
#179562=CARTESIAN_POINT('Origin',(-18.5675364832709,-75.,72.98888938658));
#179563=CARTESIAN_POINT('',(-18.5675364839017,-89.5,66.2250147575048));
#179564=CARTESIAN_POINT('Ctrl Pts',(-18.5675364848006,-89.5,79.7527640151868));
#179565=CARTESIAN_POINT('Ctrl Pts',(-15.7081614801611,-89.5,72.9888893866029));
#179566=CARTESIAN_POINT('Ctrl Pts',(-18.5675364847769,-89.5,66.2250147580291));
#179567=CARTESIAN_POINT('',(-18.5675364838598,-88.1076872567063,63.8134583461935));
#179568=CARTESIAN_POINT('Origin',(-18.5675364832709,-75.,72.98888938658));
#179569=CARTESIAN_POINT('',(-18.5675364838782,-76.3923127432566,57.0495837171963));
#179570=CARTESIAN_POINT('Ctrl Pts',(-18.5675364847385,-88.107687256259,
63.8134583459349));
#179571=CARTESIAN_POINT('Ctrl Pts',(-15.7081614801806,-82.249999999954,
60.4315210316784));
#179572=CARTESIAN_POINT('Ctrl Pts',(-18.5675364847938,-76.3923127436288,
57.0495837174103));
#179573=CARTESIAN_POINT('',(-18.5675364848006,-75.,56.9888893868452));
#179574=CARTESIAN_POINT('Origin',(-18.5675364832709,-75.,72.98888938658));
#179575=CARTESIAN_POINT('',(-16.5675364823734,-75.,58.9888893856825));
#179576=CARTESIAN_POINT('',(-17.5675364832709,-75.,57.98888938658));
#179577=CARTESIAN_POINT('Origin',(-16.5675364832709,-75.,72.98888938658));
#179578=CARTESIAN_POINT('',(-18.5675364838598,-73.6076872567056,57.0495837172181));
#179579=CARTESIAN_POINT('Origin',(-18.5675364832709,-75.,72.98888938658));
#179580=CARTESIAN_POINT('',(-18.5675364838783,-61.892312743256,63.8134583462153));
#179581=CARTESIAN_POINT('Ctrl Pts',(-18.5675364847385,-73.6076872562579,
57.0495837174757));
#179582=CARTESIAN_POINT('Ctrl Pts',(-15.7081614801806,-67.7499999999529,
60.4315210317322));
#179583=CARTESIAN_POINT('Ctrl Pts',(-18.5675364847938,-61.8923127436277,
63.8134583460004));
#179584=CARTESIAN_POINT('Origin',(-18.5675364832709,-75.,72.98888938658));
#179585=CARTESIAN_POINT('Origin',(-31.5405364832709,-75.,72.98888938658));
#179586=CARTESIAN_POINT('',(-27.5675364832709,-73.60768725693,57.04958371709));
#179587=CARTESIAN_POINT('',(-27.5675364832709,-76.39231274307,57.04958371709));
#179588=CARTESIAN_POINT('Origin',(-16.5675364832709,-75.,89.73204719308));
#179589=CARTESIAN_POINT('',(-27.5675364832709,-73.60768725693,88.92819505607));
#179590=CARTESIAN_POINT('',(-27.5675364832709,-61.89231274307,82.164320426837));
#179591=CARTESIAN_POINT('Origin',(-16.5675364832709,-75.,56.24573158008));
#179592=CARTESIAN_POINT('',(-27.5675364832709,-88.10768725693,63.813458346323));
#179593=CARTESIAN_POINT('Origin',(-16.5675364832709,-60.5,64.61731048333));
#179594=CARTESIAN_POINT('',(-27.5675364832709,-61.89231274307,63.813458346323));
#179595=CARTESIAN_POINT('Origin',(-31.5405364832709,-75.,72.98888938658));
#179596=CARTESIAN_POINT('',(-27.5675364832709,-89.5,66.225014757346));
#179597=CARTESIAN_POINT('Origin',(-31.5405364832709,-75.,72.98888938658));
#179598=CARTESIAN_POINT('',(-27.5675364832709,-60.5,66.225014757346));
#179599=CARTESIAN_POINT('Origin',(-16.5675364832709,-60.5,81.36046828983));
#179600=CARTESIAN_POINT('',(-27.5675364832709,-60.5,79.752764015814));
#179601=CARTESIAN_POINT('Origin',(-16.5675364832709,-89.5,81.36046828983));
#179602=CARTESIAN_POINT('',(-27.5675364832709,-88.10768725693,82.164320426837));
#179603=CARTESIAN_POINT('',(-27.5675364832709,-76.39231274307,88.92819505607));
#179604=CARTESIAN_POINT('Origin',(-31.5405364832709,-75.,72.98888938658));
#179605=CARTESIAN_POINT('Origin',(-31.5405364832709,-75.,72.98888938658));
#179606=CARTESIAN_POINT('',(-27.5675364832709,-89.5,79.752764015814));
#179607=CARTESIAN_POINT('Origin',(-31.5405364832709,-75.,72.98888938658));
#179608=CARTESIAN_POINT('Origin',(-16.5675364832709,-89.5,64.61731048333));
#179609=CARTESIAN_POINT('Origin',(-29.5675364832709,-75.,72.98888938658));
#179610=CARTESIAN_POINT('Ctrl Pts',(-29.4235335827009,-87.55585084311,76.731819067654));
#179611=CARTESIAN_POINT('Ctrl Pts',(-29.3785752787509,-88.14324409162,74.761378091484));
#179612=CARTESIAN_POINT('Ctrl Pts',(-29.2886586708509,-88.3725131074,70.540717962258));
#179613=CARTESIAN_POINT('Ctrl Pts',(-29.1537837590009,-85.80712443056,64.740945094149));
#179614=CARTESIAN_POINT('Ctrl Pts',(-29.0189088471409,-80.89008803912,60.73624495104));
#179615=CARTESIAN_POINT('Ctrl Pts',(-28.8840339352909,-74.691455216807,
59.3974994093));
#179616=CARTESIAN_POINT('Ctrl Pts',(-28.7491590234309,-68.559950359161,
61.01614190121));
#179617=CARTESIAN_POINT('Ctrl Pts',(-28.6142841115809,-63.82974243489,65.239934789744));
#179618=CARTESIAN_POINT('Ctrl Pts',(-28.4794091997309,-61.53007762407,71.14982987547));
#179619=CARTESIAN_POINT('Ctrl Pts',(-28.3445342878709,-62.1613422859,77.459886586808));
#179620=CARTESIAN_POINT('Ctrl Pts',(-28.2096593760209,-65.586178918236,
82.797096210383));
#179621=CARTESIAN_POINT('Ctrl Pts',(-28.0747844641709,-71.059375111067,
86.00013159165));
#179622=CARTESIAN_POINT('Ctrl Pts',(-27.9399095523109,-77.390014473847,
86.37204219574));
#179623=CARTESIAN_POINT('Ctrl Pts',(-27.8050346404609,-83.200609009059,
83.83190373521));
#179624=CARTESIAN_POINT('Ctrl Pts',(-27.6701597286009,-87.22682761174,78.932426619492));
#179625=CARTESIAN_POINT('Ctrl Pts',(-27.5352848167509,-88.59260271637,72.7396913102611));
#179626=CARTESIAN_POINT('Ctrl Pts',(-27.4004099049009,-87.00075441549,66.601179175152));
#179627=CARTESIAN_POINT('Ctrl Pts',(-27.2655349930409,-82.797654032634,
61.8525731252));
#179628=CARTESIAN_POINT('Ctrl Pts',(-27.1306600811909,-76.897856957019,
59.52712548816));
#179629=CARTESIAN_POINT('Ctrl Pts',(-26.9957851693409,-70.585103932253,
60.13083195176));
#179630=CARTESIAN_POINT('Ctrl Pts',(-26.8609102574809,-65.232991059679,
63.532331627755));
#179631=CARTESIAN_POINT('Ctrl Pts',(-26.7260353456309,-62.00608811552,68.991489954176));
#179632=CARTESIAN_POINT('Ctrl Pts',(-26.5911604337809,-61.60653904254,75.320445064586));
#179633=CARTESIAN_POINT('Ctrl Pts',(-26.4562855219229,-64.12128199053,81.142075432836));
#179634=CARTESIAN_POINT('Ctrl Pts',(-26.3214106100699,-69.003132368767,
85.18964866916));
#179635=CARTESIAN_POINT('Ctrl Pts',(-26.1865356982159,-75.1898451699075,
86.58245060783));
#179636=CARTESIAN_POINT('Ctrl Pts',(-26.0516607863629,-81.33524931199,85.01742067074));
#179637=CARTESIAN_POINT('Ctrl Pts',(-25.9167858745089,-86.10216283013,80.835094323236));
#179638=CARTESIAN_POINT('Ctrl Pts',(-25.7819109626559,-88.45334768832,74.945508333151));
#179639=CARTESIAN_POINT('Ctrl Pts',(-25.6470360508029,-87.87721613395,68.630175581195));
#179640=CARTESIAN_POINT('Ctrl Pts',(-25.5121611389499,-84.499098730494,
63.263275982751));
#179641=CARTESIAN_POINT('Ctrl Pts',(-25.3772862270959,-79.054155289863,
60.01251283554));
#179642=CARTESIAN_POINT('Ctrl Pts',(-25.2424113152429,-72.726732877904,
59.58553507798));
#179643=CARTESIAN_POINT('Ctrl Pts',(-25.1524947073409,-68.839040027706,
61.24456506882));
#179644=CARTESIAN_POINT('Ctrl Pts',(-25.1075364033899,-67.188343111843,
62.4704803028));
#179645=CARTESIAN_POINT('Ctrl Pts',(-29.5803515522709,-87.26716059124,76.645759801271));
#179646=CARTESIAN_POINT('Ctrl Pts',(-29.5353932483209,-87.84104820744,74.720624165918));
#179647=CARTESIAN_POINT('Ctrl Pts',(-29.4454766404109,-88.06504575808,70.597007514748));
#179648=CARTESIAN_POINT('Ctrl Pts',(-29.3106017285609,-85.55864175003,64.930585855648));
#179649=CARTESIAN_POINT('Ctrl Pts',(-29.1757268167109,-80.754660259608,
61.01796373317));
#179650=CARTESIAN_POINT('Ctrl Pts',(-29.0408519048509,-74.698549429079,
59.70999928245));
#179651=CARTESIAN_POINT('Ctrl Pts',(-28.9059769930009,-68.708023124285,
61.29142515603));
#179652=CARTESIAN_POINT('Ctrl Pts',(-28.7711020811409,-64.08657444972,65.418102536579));
#179653=CARTESIAN_POINT('Ctrl Pts',(-28.6362271692909,-61.83978465483,71.192114429511));
#179654=CARTESIAN_POINT('Ctrl Pts',(-28.5013522574409,-62.4565349714,77.357087236615));
#179655=CARTESIAN_POINT('Ctrl Pts',(-28.3664773455809,-65.802626088017,
82.571581131104));
#179656=CARTESIAN_POINT('Ctrl Pts',(-28.2316024337309,-71.149979882179,
85.70097075929));
#179657=CARTESIAN_POINT('Ctrl Pts',(-28.0967275218809,-77.335062094356,
86.06433021321));
#179658=CARTESIAN_POINT('Ctrl Pts',(-27.9618526100209,-83.012056603505,
83.58259585616));
#179659=CARTESIAN_POINT('Ctrl Pts',(-27.8269776981709,-86.94570242263,78.795769910022));
#179660=CARTESIAN_POINT('Ctrl Pts',(-27.6921027863109,-88.28007495933,72.7454209940753));
#179661=CARTESIAN_POINT('Ctrl Pts',(-27.5572278744609,-86.72482721166,66.748048526563));
#179662=CARTESIAN_POINT('Ctrl Pts',(-27.4223529626109,-82.618366564596,
62.108624745));
#179663=CARTESIAN_POINT('Ctrl Pts',(-27.2874780507509,-76.854220503396,
59.83664493523));
#179664=CARTESIAN_POINT('Ctrl Pts',(-27.1526031389009,-70.68661337782,60.42647068511));
#179665=CARTESIAN_POINT('Ctrl Pts',(-27.0177282270509,-65.457558897109,
63.749761420078));
#179666=CARTESIAN_POINT('Ctrl Pts',(-26.8828533151909,-62.30485048069,69.083400113308));
#179667=CARTESIAN_POINT('Ctrl Pts',(-26.7479784033409,-61.91448803505,75.266836798267));
#179668=CARTESIAN_POINT('Ctrl Pts',(-26.6131034914909,-64.37141078558,80.954613399192));
#179669=CARTESIAN_POINT('Ctrl Pts',(-26.4782285796339,-69.141015276789,
84.90912285579));
#179670=CARTESIAN_POINT('Ctrl Pts',(-26.3433536677799,-75.1854801570906,
86.26990081237));
#179671=CARTESIAN_POINT('Ctrl Pts',(-26.2084787559269,-81.189586167187,
84.74085480758));
#179672=CARTESIAN_POINT('Ctrl Pts',(-26.0736038440729,-85.84689648269,80.654690549114));
#179673=CARTESIAN_POINT('Ctrl Pts',(-25.9387289322199,-88.14402175087,74.900520795182));
#179674=CARTESIAN_POINT('Ctrl Pts',(-25.8038540203669,-87.58113689443,68.730393256763));
#179675=CARTESIAN_POINT('Ctrl Pts',(-25.6689791085129,-84.280690815386,
63.486892033801));
#179676=CARTESIAN_POINT('Ctrl Pts',(-25.5341041966599,-78.960940172354,
60.31087201977));
#179677=CARTESIAN_POINT('Ctrl Pts',(-25.3992292848069,-72.779000945297,
59.89371154324));
#179678=CARTESIAN_POINT('Ctrl Pts',(-25.3093126769049,-68.980695826933,
61.51459630666));
#179679=CARTESIAN_POINT('Ctrl Pts',(-25.2643543729539,-67.367952540366,
62.71232469914));
#179680=CARTESIAN_POINT('Ctrl Pts',(-29.7371695218309,-86.97847033937,76.559700534901));
#179681=CARTESIAN_POINT('Ctrl Pts',(-29.6922112178809,-87.53885232326,74.679870240367));
#179682=CARTESIAN_POINT('Ctrl Pts',(-29.6022946099809,-87.75757840877,70.653297067253));
#179683=CARTESIAN_POINT('Ctrl Pts',(-29.4674196981209,-85.31015906951,65.120226617163));
#179684=CARTESIAN_POINT('Ctrl Pts',(-29.3325447862709,-80.619232480115,
61.29968251531));
#179685=CARTESIAN_POINT('Ctrl Pts',(-29.1976698744209,-74.7056436413761,
60.02249915561));
#179686=CARTESIAN_POINT('Ctrl Pts',(-29.0627949625609,-68.856095889434,
61.56670841083));
#179687=CARTESIAN_POINT('Ctrl Pts',(-28.9279200507109,-64.34340646456,65.596270283389));
#179688=CARTESIAN_POINT('Ctrl Pts',(-28.7930451388509,-62.1494916856,71.23439898352));
#179689=CARTESIAN_POINT('Ctrl Pts',(-28.6581702270009,-62.75172765689,77.254287886388));
#179690=CARTESIAN_POINT('Ctrl Pts',(-28.5232953151509,-66.01907325777,82.346066051798));
#179691=CARTESIAN_POINT('Ctrl Pts',(-28.3884204032909,-71.240584653253,
85.40180992691));
#179692=CARTESIAN_POINT('Ctrl Pts',(-28.2535454914409,-77.280109714823,
85.75661823069));
#179693=CARTESIAN_POINT('Ctrl Pts',(-28.1186705795909,-82.823504197914,
83.33328797713));
#179694=CARTESIAN_POINT('Ctrl Pts',(-27.9837956677309,-86.66457723349,78.659113200594));
#179695=CARTESIAN_POINT('Ctrl Pts',(-27.8489207558809,-87.96754720229,72.7511506779378));
#179696=CARTESIAN_POINT('Ctrl Pts',(-27.7140458440209,-86.44890000785,66.894917878018));
#179697=CARTESIAN_POINT('Ctrl Pts',(-27.5791709321709,-82.439079096599,
62.36467636483));
#179698=CARTESIAN_POINT('Ctrl Pts',(-27.4442960203209,-76.810584049825,
60.1461643823));
#179699=CARTESIAN_POINT('Ctrl Pts',(-27.3094211084609,-70.788122823435,
60.72210941845));
#179700=CARTESIAN_POINT('Ctrl Pts',(-27.1745461966109,-65.682126734574,
63.967191212364));
#179701=CARTESIAN_POINT('Ctrl Pts',(-27.0396712847609,-62.60361284588,69.175310272392));
#179702=CARTESIAN_POINT('Ctrl Pts',(-26.9047963729009,-62.22243702755,75.213228531899));
#179703=CARTESIAN_POINT('Ctrl Pts',(-26.7699214610509,-64.6215395806,80.767151365512));
#179704=CARTESIAN_POINT('Ctrl Pts',(-26.6350465492009,-69.27889818477,84.62859704241));
#179705=CARTESIAN_POINT('Ctrl Pts',(-26.5001716373439,-75.1811151442317,
85.95735101692));
#179706=CARTESIAN_POINT('Ctrl Pts',(-26.3652967254909,-81.043923022351,
84.46428894445));
#179707=CARTESIAN_POINT('Ctrl Pts',(-26.2304218136369,-85.59163013523,80.47428677502));
#179708=CARTESIAN_POINT('Ctrl Pts',(-26.0955469017839,-87.83469581341,74.855533257242));
#179709=CARTESIAN_POINT('Ctrl Pts',(-25.9606719899309,-87.28505765493,68.830610932353));
#179710=CARTESIAN_POINT('Ctrl Pts',(-25.8257970780769,-84.062282900292,
63.710508084863));
#179711=CARTESIAN_POINT('Ctrl Pts',(-25.6909221662239,-78.867725054857,
60.609231204));
#179712=CARTESIAN_POINT('Ctrl Pts',(-25.5560472543709,-72.831269012692,
60.20188800851));
#179713=CARTESIAN_POINT('Ctrl Pts',(-25.4661306464689,-69.122351626158,
61.7846275445));
#179714=CARTESIAN_POINT('Ctrl Pts',(-25.4211723425179,-67.547561968885,
62.95416909548));
#179715=CARTESIAN_POINT('Ctrl Pts',(-29.8939874914009,-86.6897800875,76.473641268518));
#179716=CARTESIAN_POINT('Ctrl Pts',(-29.8490291874409,-87.23665643908,74.639116314802));
#179717=CARTESIAN_POINT('Ctrl Pts',(-29.7591125795409,-87.45011105946,70.709586619743));
#179718=CARTESIAN_POINT('Ctrl Pts',(-29.6242376676909,-85.06167638898,65.309867378662));
#179719=CARTESIAN_POINT('Ctrl Pts',(-29.4893627558309,-80.483804700603,
61.58140129744));
#179720=CARTESIAN_POINT('Ctrl Pts',(-29.3544878439809,-74.7127378536479,
60.33499902876));
#179721=CARTESIAN_POINT('Ctrl Pts',(-29.2196129321309,-69.004168654558,
61.84199166565));
#179722=CARTESIAN_POINT('Ctrl Pts',(-29.0847380202709,-64.60023847939,65.774438030224));
#179723=CARTESIAN_POINT('Ctrl Pts',(-28.9498631084209,-62.45919871637,71.276683537561));
#179724=CARTESIAN_POINT('Ctrl Pts',(-28.8149881965709,-63.04692034239,77.151488536196));
#179725=CARTESIAN_POINT('Ctrl Pts',(-28.6801132847109,-66.235520427551,
82.120550972519));
#179726=CARTESIAN_POINT('Ctrl Pts',(-28.5452383728609,-71.331189424365,
85.10264909454));
#179727=CARTESIAN_POINT('Ctrl Pts',(-28.4103634610009,-77.225157335332,
85.44890624816));
#179728=CARTESIAN_POINT('Ctrl Pts',(-28.2754885491509,-82.634951792361,
83.08398009808));
#179729=CARTESIAN_POINT('Ctrl Pts',(-28.1406136373009,-86.38345204438,78.522456491124));
#179730=CARTESIAN_POINT('Ctrl Pts',(-28.0057387254409,-87.65501944525,72.7568803617516));
#179731=CARTESIAN_POINT('Ctrl Pts',(-27.8708638135909,-86.17297280402,67.041787229428));
#179732=CARTESIAN_POINT('Ctrl Pts',(-27.7359889017409,-82.259791628561,
62.62072798463));
#179733=CARTESIAN_POINT('Ctrl Pts',(-27.6011139898809,-76.766947596202,
60.45568382937));
#179734=CARTESIAN_POINT('Ctrl Pts',(-27.4662390780309,-70.889632269001,
61.0177481518));
#179735=CARTESIAN_POINT('Ctrl Pts',(-27.3313641661709,-65.906694572004,
64.184621004688));
#179736=CARTESIAN_POINT('Ctrl Pts',(-27.1964892543209,-62.90237521105,69.267220431524));
#179737=CARTESIAN_POINT('Ctrl Pts',(-27.0616143424709,-62.53038602006,75.159620265581));
#179738=CARTESIAN_POINT('Ctrl Pts',(-26.9267394306109,-64.87166837565,80.579689331869));
#179739=CARTESIAN_POINT('Ctrl Pts',(-26.7918645187609,-69.416781092793,
84.34807122905));
#179740=CARTESIAN_POINT('Ctrl Pts',(-26.6569896069109,-75.1767501314152,
85.64480122147));
#179741=CARTESIAN_POINT('Ctrl Pts',(-26.5221146950539,-80.898259877549,
84.18772308129));
#179742=CARTESIAN_POINT('Ctrl Pts',(-26.3872397832009,-85.3363637878,80.293883000897));
#179743=CARTESIAN_POINT('Ctrl Pts',(-26.2523648713479,-87.52536987595,74.810545719273));
#179744=CARTESIAN_POINT('Ctrl Pts',(-26.1174899594939,-86.98897841541,68.93082860792));
#179745=CARTESIAN_POINT('Ctrl Pts',(-25.9826150476409,-83.843874985184,
63.934124135913));
#179746=CARTESIAN_POINT('Ctrl Pts',(-25.8477401357879,-78.774509937348,
60.90759038823));
#179747=CARTESIAN_POINT('Ctrl Pts',(-25.7128652239349,-72.883537080085,
60.51006447377));
#179748=CARTESIAN_POINT('Ctrl Pts',(-25.6229486160329,-69.264007425385,
62.05465878235));
#179749=CARTESIAN_POINT('Ctrl Pts',(-25.5779903120819,-67.727171397409,
63.196013491817));
#179750=CARTESIAN_POINT('Ctrl Pts',(-29.3659074908668,-88.0481395961661,
72.910724257937));
#179751=CARTESIAN_POINT('Ctrl Pts',(-29.3564982338821,-88.0460045428066,
72.4863077063651));
#179752=CARTESIAN_POINT('Ctrl Pts',(-29.3471083831415,-88.0232803767141,
72.061989631977));
#179753=CARTESIAN_POINT('Ctrl Pts',(-29.3281064149641,-87.934573512206,
71.2015622468502));
#179754=CARTESIAN_POINT('Ctrl Pts',(-29.3185886995406,-87.8671769059716,
70.7675430526915));
#179755=CARTESIAN_POINT('Ctrl Pts',(-29.2896717560233,-87.5960608923731,
69.4669196523705));
#179756=CARTESIAN_POINT('Ctrl Pts',(-29.2702173424168,-87.3252271347852,
68.6164798142884));
#179757=CARTESIAN_POINT('Ctrl Pts',(-29.2253010143824,-86.5131076515063,
66.742024930945));
#179758=CARTESIAN_POINT('Ctrl Pts',(-29.1996910935634,-85.9137974945729,
65.7401241308678));
#179759=CARTESIAN_POINT('Ctrl Pts',(-29.1554746269511,-84.6578977939495,
64.1717373950071));
#179760=CARTESIAN_POINT('Ctrl Pts',(-29.1369985236878,-84.0611558696511,
63.5616725854627));
#179761=CARTESIAN_POINT('Ctrl Pts',(-29.0982964749951,-82.7026349825422,
62.4171369804774));
#179762=CARTESIAN_POINT('Ctrl Pts',(-29.0780486887075,-81.9304516311765,
61.8944315877894));
#179763=CARTESIAN_POINT('Ctrl Pts',(-29.0439061828359,-80.5727347676091,
61.1728735765531));
#179764=CARTESIAN_POINT('Ctrl Pts',(-29.0302053743383,-80.0156938632889,
60.9255547302426));
#179765=CARTESIAN_POINT('Ctrl Pts',(-29.0050768977302,-78.9391594068913,
60.537100991496));
#179766=CARTESIAN_POINT('Ctrl Pts',(-28.9935432067017,-78.4270849802294,
60.3872937961839));
#179767=CARTESIAN_POINT('Ctrl Pts',(-28.9678777664002,-77.2694113129645,
60.1235667201636));
#179768=CARTESIAN_POINT('Ctrl Pts',(-28.9537517745064,-76.6200096747148,
60.0257507510677));
#179769=CARTESIAN_POINT('Ctrl Pts',(-28.9272328280987,-75.4132633020343,
59.93509232377));
#179770=CARTESIAN_POINT('Ctrl Pts',(-28.9148503310648,-74.8568225856496,
59.9285568053376));
#179771=CARTESIAN_POINT('Ctrl Pts',(-28.8942428497637,-73.9467752421308,
59.9765772975495));
#179772=CARTESIAN_POINT('Ctrl Pts',(-28.8862407188741,-73.5930365781412,
60.0099924734182));
#179773=CARTESIAN_POINT('Ctrl Pts',(-28.8628376106062,-72.5429562198852,
60.1535934566403));
#179774=CARTESIAN_POINT('Ctrl Pts',(-28.8477724295467,-71.8538171714245,
60.3060433724034));
#179775=CARTESIAN_POINT('Ctrl Pts',(-28.8184383628547,-70.5459349980751,
60.7072179776806));
#179776=CARTESIAN_POINT('Ctrl Pts',(-28.8041619638653,-69.9252544251782,
60.9501893074854));
#179777=CARTESIAN_POINT('Ctrl Pts',(-28.7788113746183,-68.8929646488808,
61.4474152891473));
#179778=CARTESIAN_POINT('Ctrl Pts',(-28.767835471829,-68.4708619183447,
61.6801004622464));
#179779=CARTESIAN_POINT('Ctrl Pts',(-28.7507664251534,-67.8354245741352,
62.0782315790565));
#179780=CARTESIAN_POINT('Ctrl Pts',(-28.7446895251965,-67.6123225281541,
62.2279161008187));
#179781=CARTESIAN_POINT('Ctrl Pts',(-28.7305582988274,-67.0953388264515,
62.5990202479308));
#179782=CARTESIAN_POINT('Ctrl Pts',(-28.7225808515193,-66.8062336479153,
62.8259709421714));
#179783=CARTESIAN_POINT('Ctrl Pts',(-28.7013578651677,-66.0558928438563,
63.4680002526907));
#179784=CARTESIAN_POINT('Ctrl Pts',(-28.6882686874363,-65.6133280976073,
63.9049486073402));
#179785=CARTESIAN_POINT('Ctrl Pts',(-28.6666858385585,-64.9489264935309,
64.6603239558346));
#179786=CARTESIAN_POINT('Ctrl Pts',(-28.6583249823005,-64.7068801937676,
64.9611121847821));
#179787=CARTESIAN_POINT('Ctrl Pts',(-28.6410882123786,-64.2464948877883,
65.5877306343096));
#179788=CARTESIAN_POINT('Ctrl Pts',(-28.6321488163013,-64.0285887231609,
65.9138981003384));
#179789=CARTESIAN_POINT('Ctrl Pts',(-28.6167537023254,-63.680887421671,
66.4890168565324));
#179790=CARTESIAN_POINT('Ctrl Pts',(-28.610328827005,-63.5436822219399,
66.7334806652167));
#179791=CARTESIAN_POINT('Ctrl Pts',(-28.5984854221818,-63.3019585873584,
67.1993026659102));
#179792=CARTESIAN_POINT('Ctrl Pts',(-28.5930704079703,-63.1957781442392,
67.419153535765));
#179793=CARTESIAN_POINT('Ctrl Pts',(-28.576222129306,-62.8802537249818,
68.1228949558838));
#179794=CARTESIAN_POINT('Ctrl Pts',(-28.5650682955872,-62.6941578388861,
68.6170188276551));
#179795=CARTESIAN_POINT('Ctrl Pts',(-28.545793745091,-62.4247797613169,
69.4876004126718));
#179796=CARTESIAN_POINT('Ctrl Pts',(-28.5376684957557,-62.3272961663442,
69.8596880564267));
#179797=CARTESIAN_POINT('Ctrl Pts',(-28.523233234306,-62.1855983227819,
70.5161434091827));
#179798=CARTESIAN_POINT('Ctrl Pts',(-28.5169819108951,-62.1341452449762,
70.7989808731062));
#179799=CARTESIAN_POINT('Ctrl Pts',(-28.4996699074065,-62.0197648406076,
71.5701861668623));
#179800=CARTESIAN_POINT('Ctrl Pts',(-28.4882982896073,-61.9748410256592,
72.0612406787676));
#179801=CARTESIAN_POINT('Ctrl Pts',(-28.471322229869,-61.9493875669456,
72.8005829324056));
#179802=CARTESIAN_POINT('Ctrl Pts',(-28.465664165641,-61.9479446733414,
73.0481500053425));
#179803=CARTESIAN_POINT('Ctrl Pts',(-28.4551716019025,-61.9587112129092,
73.5141902924898));
#179804=CARTESIAN_POINT('Ctrl Pts',(-28.4503395173441,-61.9693462642277,
73.7321878396621));
#179805=CARTESIAN_POINT('Ctrl Pts',(-28.4334128965999,-62.0269819057531,
74.5067571199237));
#179806=CARTESIAN_POINT('Ctrl Pts',(-28.4217088175756,-62.1046530214977,
75.0606813516689));
#179807=CARTESIAN_POINT('Ctrl Pts',(-28.4001844763301,-62.3107848251598,
76.0622387749575));
#179808=CARTESIAN_POINT('Ctrl Pts',(-28.3903752305105,-62.4285150974339,
76.5121139327343));
#179809=CARTESIAN_POINT('Ctrl Pts',(-28.3753344049142,-62.6379884110952,
77.1690374466618));
#179810=CARTESIAN_POINT('Ctrl Pts',(-28.3703383053425,-62.7118876037204,
77.3818208990407));
#179811=CARTESIAN_POINT('Ctrl Pts',(-28.3539567178157,-62.9679285208451,
78.0622418099726));
#179812=CARTESIAN_POINT('Ctrl Pts',(-28.3423086960805,-63.171521881072,
78.5218357355849));
#179813=CARTESIAN_POINT('Ctrl Pts',(-28.3257320578495,-63.5029030303266,
79.1662560371414));
#179814=CARTESIAN_POINT('Ctrl Pts',(-28.3206683556837,-63.6099001836908,
79.361775026428));
#179815=CARTESIAN_POINT('Ctrl Pts',(-28.311078153775,-63.8253072023904,
79.7321578643301));
#179816=CARTESIAN_POINT('Ctrl Pts',(-28.3065585803607,-63.9327431373142,
79.9070518827553));
#179817=CARTESIAN_POINT('Ctrl Pts',(-28.2903497084108,-64.3393885356207,
80.5346700381858));
#179818=CARTESIAN_POINT('Ctrl Pts',(-28.2790534863171,-64.6630411220953,
80.9710469608496));
#179819=CARTESIAN_POINT('Ctrl Pts',(-28.2617405540121,-65.1944127705644,
81.601837070945));
#179820=CARTESIAN_POINT('Ctrl Pts',(-28.2557863532672,-65.3834042483339,
81.8120284013624));
#179821=CARTESIAN_POINT('Ctrl Pts',(-28.2449075332595,-65.7347911648844,
82.1784473992999));
#179822=CARTESIAN_POINT('Ctrl Pts',(-28.2400168919111,-65.8948037059415,
82.3369738580753));
#179823=CARTESIAN_POINT('Ctrl Pts',(-28.2223958775441,-66.4743186188951,
82.8824448042067));
#179824=CARTESIAN_POINT('Ctrl Pts',(-28.2092075889706,-66.9152856827901,
83.2466708682746));
#179825=CARTESIAN_POINT('Ctrl Pts',(-28.1898112960037,-67.6013903950775,
83.7415470281434));
#179826=CARTESIAN_POINT('Ctrl Pts',(-28.1835238641599,-67.8297555272949,
83.8955205339695));
#179827=CARTESIAN_POINT('Ctrl Pts',(-28.1724260254509,-68.2475777068703,
84.1581830724215));
#179828=CARTESIAN_POINT('Ctrl Pts',(-28.1675783567341,-68.4353760998163,
84.2696982570266));
#179829=CARTESIAN_POINT('Ctrl Pts',(-28.149958700384,-69.1415449055238,
84.664823071593));
#179830=CARTESIAN_POINT('Ctrl Pts',(-28.1377313668127,-69.6768672641444,
84.9174692290254));
#179831=CARTESIAN_POINT('Ctrl Pts',(-28.1201770297299,-70.455680847885,
85.2226728581861));
#179832=CARTESIAN_POINT('Ctrl Pts',(-28.1149880895017,-70.6871188022322,
85.3059418428659));
#179833=CARTESIAN_POINT('Ctrl Pts',(-28.1050279728183,-71.1281712184913,
85.4508261624183));
#179834=CARTESIAN_POINT('Ctrl Pts',(-28.1002660044092,-71.3373373300875,
85.5138227899195));
#179835=CARTESIAN_POINT('Ctrl Pts',(-28.0843589237699,-72.0294388552241,
85.7036742906909));
#179836=CARTESIAN_POINT('Ctrl Pts',(-28.0729223312909,-72.5184809261174,
85.8084453254484));
#179837=CARTESIAN_POINT('Ctrl Pts',(-28.050883270265,-73.4700006659628,
85.9561309750036));
#179838=CARTESIAN_POINT('Ctrl Pts',(-28.0402809736981,-73.9319196816796,
86.0029343223826));
#179839=CARTESIAN_POINT('Ctrl Pts',(-28.0252281645065,-74.609077915433,
86.0347769534915));
#179840=CARTESIAN_POINT('Ctrl Pts',(-28.0205423787538,-74.8232630500173,
86.0394917038328));
#179841=CARTESIAN_POINT('Ctrl Pts',(-28.0070172334021,-75.4524680389126,
86.0374732751357));
#179842=CARTESIAN_POINT('Ctrl Pts',(-27.9983748948768,-75.8669829436328,
86.0160201738747));
#179843=CARTESIAN_POINT('Ctrl Pts',(-27.9842063416296,-76.5401689750176,
85.9489422436268));
#179844=CARTESIAN_POINT('Ctrl Pts',(-27.9787046285364,-76.8000028522898,
85.9151310849484));
#179845=CARTESIAN_POINT('Ctrl Pts',(-27.9680786331094,-77.2910612907271,
85.8362548589024));
#179846=CARTESIAN_POINT('Ctrl Pts',(-27.9629597312461,-77.5225283259899,
85.7926708694011));
#179847=CARTESIAN_POINT('Ctrl Pts',(-27.9459079923068,-78.2773135689571,
85.6295219742758));
#179848=CARTESIAN_POINT('Ctrl Pts',(-27.9336692048689,-78.7951050754462,
85.4840841657931));
#179849=CARTESIAN_POINT('Ctrl Pts',(-27.9131107193046,-79.6471742861783,
85.1874098991876));
#179850=CARTESIAN_POINT('Ctrl Pts',(-27.9047868360306,-79.9873185335186,
85.0528224331465));
#179851=CARTESIAN_POINT('Ctrl Pts',(-27.8904074150385,-80.5730290701081,
84.7919520042867));
#179852=CARTESIAN_POINT('Ctrl Pts',(-27.8842971545009,-80.8212953221514,
84.6717539991534));
#179853=CARTESIAN_POINT('Ctrl Pts',(-27.8698641651539,-81.4097433606845,
84.3630061942767));
#179854=CARTESIAN_POINT('Ctrl Pts',(-27.861710200252,-81.7452306837839,
84.166903060444));
#179855=CARTESIAN_POINT('Ctrl Pts',(-27.8453550084117,-82.3999208736734,
83.743847470235));
#179856=CARTESIAN_POINT('Ctrl Pts',(-27.8371328291244,-82.7192165073017,
83.5164356111363));
#179857=CARTESIAN_POINT('Ctrl Pts',(-27.8216158902492,-83.2835271823475,
83.0752714525562));
#179858=CARTESIAN_POINT('Ctrl Pts',(-27.8144342767874,-83.5319170271531,
82.8658224661742));
#179859=CARTESIAN_POINT('Ctrl Pts',(-27.7925141076131,-84.2572804367664,
82.2069105176513));
#179860=CARTESIAN_POINT('Ctrl Pts',(-27.7775244449214,-84.7095831907395,
81.7301117026834));
#179861=CARTESIAN_POINT('Ctrl Pts',(-27.7543237430217,-85.3612165647386,
80.9306647300642));
#179862=CARTESIAN_POINT('Ctrl Pts',(-27.7459456038675,-85.5862339849805,
80.6288772514887));
#179863=CARTESIAN_POINT('Ctrl Pts',(-27.7285710578544,-86.034427501779,
79.9691890098338));
#179864=CARTESIAN_POINT('Ctrl Pts',(-27.7197240144229,-86.2532168953495,
79.6100593961399));
#179865=CARTESIAN_POINT('Ctrl Pts',(-27.7023250909202,-86.6476929956993,
78.8856638739585));
#179866=CARTESIAN_POINT('Ctrl Pts',(-27.6936986564007,-86.8246641272642,
78.52105954023));
#179867=CARTESIAN_POINT('Ctrl Pts',(-27.6675797083516,-87.2965186957519,
77.4225764407828));
#179868=CARTESIAN_POINT('Ctrl Pts',(-27.6496751030241,-87.5431103114704,
76.6677537942569));
#179869=CARTESIAN_POINT('Ctrl Pts',(-27.6227789730324,-87.8109154077877,
75.5014481464235));
#179870=CARTESIAN_POINT('Ctrl Pts',(-27.61368927909,-87.8834238266364,75.1015430110265));
#179871=CARTESIAN_POINT('Ctrl Pts',(-27.5967623749459,-87.984714478606,
74.340769305862));
#179872=CARTESIAN_POINT('Ctrl Pts',(-27.5889116823622,-88.0174175457536,
73.9804215063339));
#179873=CARTESIAN_POINT('Ctrl Pts',(-27.5726952476485,-88.0537744436508,
73.2211702198945));
#179874=CARTESIAN_POINT('Ctrl Pts',(-27.5643023785365,-88.0543305131637,
72.8232192864537));
#179875=CARTESIAN_POINT('Ctrl Pts',(-27.5329917923186,-87.9902150124072,
71.3750406569378));
#179876=CARTESIAN_POINT('Ctrl Pts',(-27.5093033935216,-87.8166446035142,
70.3293263596883));
#179877=CARTESIAN_POINT('Ctrl Pts',(-27.4749412181969,-87.3846487974696,
68.8498644114641));
#179878=CARTESIAN_POINT('Ctrl Pts',(-27.4640850915678,-87.2212671356848,
68.387918239908));
#179879=CARTESIAN_POINT('Ctrl Pts',(-27.4356932887815,-86.7190227920006,
67.1895048707421));
#179880=CARTESIAN_POINT('Ctrl Pts',(-27.4185930823565,-86.3366767776217,
66.4766538853577));
#179881=CARTESIAN_POINT('Ctrl Pts',(-27.3825509135325,-85.4292391538904,
65.1036229345755));
#179882=CARTESIAN_POINT('Ctrl Pts',(-27.363866715291,-84.897958041126,64.4464312496957));
#179883=CARTESIAN_POINT('Ctrl Pts',(-27.3275858984294,-83.7515287572018,
63.2771098842675));
#179884=CARTESIAN_POINT('Ctrl Pts',(-27.3099850543915,-83.1410943648889,
62.7579304603558));
#179885=CARTESIAN_POINT('Ctrl Pts',(-27.2561001277643,-81.1125184247412,
61.3386319068994));
#179886=CARTESIAN_POINT('Ctrl Pts',(-27.2193312238702,-79.5515846505893,
60.6471229272152));
#179887=CARTESIAN_POINT('Ctrl Pts',(-27.163845282467,-77.1023224312657,
60.0821227070811));
#179888=CARTESIAN_POINT('Ctrl Pts',(-27.1454072056421,-76.2741375949993,
59.9740771483805));
#179889=CARTESIAN_POINT('Ctrl Pts',(-27.0942944771862,-73.9363035775581,
59.8985369954317));
#179890=CARTESIAN_POINT('Ctrl Pts',(-27.0619671031244,-72.4279016825108,
60.1092423462384));
#179891=CARTESIAN_POINT('Ctrl Pts',(-27.0204627867279,-70.6553575286048,
60.6781953554928));
#179892=CARTESIAN_POINT('Ctrl Pts',(-27.0122985285324,-70.3154085212424,
60.803211745673));
#179893=CARTESIAN_POINT('Ctrl Pts',(-26.987130500699,-69.2693881618042,
61.2394378446713));
#179894=CARTESIAN_POINT('Ctrl Pts',(-26.9704806532509,-68.5850108067239,
61.6001714360522));
#179895=CARTESIAN_POINT('Ctrl Pts',(-26.9358799470576,-67.2375402083574,
62.4688447909708));
#179896=CARTESIAN_POINT('Ctrl Pts',(-26.9179148479554,-66.5803550918046,
62.9864356224216));
#179897=CARTESIAN_POINT('Ctrl Pts',(-26.8896489617794,-65.6607017080844,
63.8646050038475));
#179898=CARTESIAN_POINT('Ctrl Pts',(-26.8796608922055,-65.35847761878,64.1837672662306));
#179899=CARTESIAN_POINT('Ctrl Pts',(-26.8613952628629,-64.8328716729229,
64.7991669455948));
#179900=CARTESIAN_POINT('Ctrl Pts',(-26.8532042088826,-64.6053354394027,
65.0903585287389));
#179901=CARTESIAN_POINT('Ctrl Pts',(-26.8358997393617,-64.1447400897498,
65.7347693972527));
#179902=CARTESIAN_POINT('Ctrl Pts',(-26.8268048243645,-63.9156848034059,
66.0908585456666));
#179903=CARTESIAN_POINT('Ctrl Pts',(-26.8007583416441,-63.3082892952384,
67.1434425427016));
#179904=CARTESIAN_POINT('Ctrl Pts',(-26.7838722948845,-62.9742535941638,
67.865720501512));
#179905=CARTESIAN_POINT('Ctrl Pts',(-26.7574958585418,-62.572988888465,
68.9894125283925));
#179906=CARTESIAN_POINT('Ctrl Pts',(-26.7484197854605,-62.4554671248045,
69.3730633903607));
#179907=CARTESIAN_POINT('Ctrl Pts',(-26.7296221149504,-62.2508872010353,
70.1712710218854));
#179908=CARTESIAN_POINT('Ctrl Pts',(-26.7199881481534,-62.1659703364768,
70.5860658314944));
#179909=CARTESIAN_POINT('Ctrl Pts',(-26.7009018638481,-62.0349643893737,
71.4411355624927));
#179910=CARTESIAN_POINT('Ctrl Pts',(-26.6914264825298,-61.9906394492088,
71.8799832795929));
#179911=CARTESIAN_POINT('Ctrl Pts',(-26.6644730958629,-61.9272184950069,
73.1416759741127));
#179912=CARTESIAN_POINT('Ctrl Pts',(-26.6471711074707,-61.9633743450345,
73.9674584135148));
#179913=CARTESIAN_POINT('Ctrl Pts',(-26.6221879434281,-62.1182970774639,
75.0896077813918));
#179914=CARTESIAN_POINT('Ctrl Pts',(-26.6152061769837,-62.1715478037406,
75.3952408793041));
#179915=CARTESIAN_POINT('Ctrl Pts',(-26.5981209290794,-62.3262333414433,
76.1278569753121));
#179916=CARTESIAN_POINT('Ctrl Pts',(-26.5879730364882,-62.4384930348096,
76.5525447979478));
#179917=CARTESIAN_POINT('Ctrl Pts',(-26.5727315788362,-62.6448972591376,
77.1974323838962));
#179918=CARTESIAN_POINT('Ctrl Pts',(-26.567469752788,-62.7237742836488,
77.4219902251026));
#179919=CARTESIAN_POINT('Ctrl Pts',(-26.5517149682415,-62.9821426894515,
78.0971663978203));
#179920=CARTESIAN_POINT('Ctrl Pts',(-26.5414479435043,-63.1810375963398,
78.5403282247619));
#179921=CARTESIAN_POINT('Ctrl Pts',(-26.5193724009043,-63.6608588511293,
79.4682464039048));
#179922=CARTESIAN_POINT('Ctrl Pts',(-26.5075648017411,-63.9497249456272,
79.9489618077733));
#179923=CARTESIAN_POINT('Ctrl Pts',(-26.4901011928254,-64.4043888612161,
80.6069925584686));
#179924=CARTESIAN_POINT('Ctrl Pts',(-26.4847749657926,-64.5463317191149,
80.8008845229701));
#179925=CARTESIAN_POINT('Ctrl Pts',(-26.4733338455652,-64.8570452251037,
81.2017922831271));
#179926=CARTESIAN_POINT('Ctrl Pts',(-26.4672136566416,-65.0270462099519,
81.4078623440487));
#179927=CARTESIAN_POINT('Ctrl Pts',(-26.4503871459154,-65.510322077725,
81.958356809343));
#179928=CARTESIAN_POINT('Ctrl Pts',(-26.4396561649183,-65.8361487294579,
82.2917405008153));
#179929=CARTESIAN_POINT('Ctrl Pts',(-26.4240726946724,-66.3536496820085,
82.7663707751346));
#179930=CARTESIAN_POINT('Ctrl Pts',(-26.4189237194656,-66.5325138718022,
82.9214875313808));
#179931=CARTESIAN_POINT('Ctrl Pts',(-26.4073473215465,-66.9492086440972,
83.2632709400261));
#179932=CARTESIAN_POINT('Ctrl Pts',(-26.4009613112974,-67.1896315259617,
83.4467584732397));
#179933=CARTESIAN_POINT('Ctrl Pts',(-26.3827457343307,-67.8953428672604,
83.9476351195622));
#179934=CARTESIAN_POINT('Ctrl Pts',(-26.3709709769733,-68.3756485690825,
84.2439355623144));
#179935=CARTESIAN_POINT('Ctrl Pts',(-26.3539767684834,-69.0667985912631,
84.6115656161261));
#179936=CARTESIAN_POINT('Ctrl Pts',(-26.349132940433,-69.2633580163022,
84.709903395342));
#179937=CARTESIAN_POINT('Ctrl Pts',(-26.338946669668,-69.6746542837514,
84.9029725362139));
#179938=CARTESIAN_POINT('Ctrl Pts',(-26.3336041872981,-69.8897244447453,
84.9970074859295));
#179939=CARTESIAN_POINT('Ctrl Pts',(-26.314231955768,-70.6735487500045,
85.3149592179739));
#179940=CARTESIAN_POINT('Ctrl Pts',(-26.3000246937031,-71.255992426112,
85.5051243484357));
#179941=CARTESIAN_POINT('Ctrl Pts',(-26.2816122099814,-72.0632443492675,
85.7060943795211));
#179942=CARTESIAN_POINT('Ctrl Pts',(-26.2768286975967,-72.2785241214213,
85.7537910136647));
#179943=CARTESIAN_POINT('Ctrl Pts',(-26.2660720341698,-72.7714956543973,
85.8498414623097));
#179944=CARTESIAN_POINT('Ctrl Pts',(-26.260134841256,-73.0499760709272,
85.8946831020152));
#179945=CARTESIAN_POINT('Ctrl Pts',(-26.2429700519115,-73.8615368526726,
85.9985253898064));
#179946=CARTESIAN_POINT('Ctrl Pts',(-26.2317986029984,-74.3976751519069,
86.0338075190741));
#179947=CARTESIAN_POINT('Ctrl Pts',(-26.2155064654886,-75.1493185610999,
86.0374428848513));
#179948=CARTESIAN_POINT('Ctrl Pts',(-26.2107555175633,-75.3647440062942,
86.0332104066427));
#179949=CARTESIAN_POINT('Ctrl Pts',(-26.2003640862362,-75.8285358965611,
86.0127296677718));
#179950=CARTESIAN_POINT('Ctrl Pts',(-26.1947077546196,-76.076831658566,
85.9947172503313));
#179951=CARTESIAN_POINT('Ctrl Pts',(-26.174118315283,-76.9727601170871,
85.9040944046082));
#179952=CARTESIAN_POINT('Ctrl Pts',(-26.1589940543832,-77.6162491189474,
85.7902962812833));
#179953=CARTESIAN_POINT('Ctrl Pts',(-26.1398650652927,-78.4544973207557,
85.575212258799));
#179954=CARTESIAN_POINT('Ctrl Pts',(-26.1352371189142,-78.6597702370693,
85.5170117907657));
#179955=CARTESIAN_POINT('Ctrl Pts',(-26.1249826697253,-79.1176792880076,
85.3747766623542));
#179956=CARTESIAN_POINT('Ctrl Pts',(-26.1193886159666,-79.36930568476,85.2879755540693));
#179957=CARTESIAN_POINT('Ctrl Pts',(-26.1032508837398,-80.0895803369744,
85.0145418610182));
#179958=CARTESIAN_POINT('Ctrl Pts',(-26.0927596236044,-80.5507285382675,
84.8081327170226));
#179959=CARTESIAN_POINT('Ctrl Pts',(-26.0768782923636,-81.2019710439065,
84.4706061229787));
#179960=CARTESIAN_POINT('Ctrl Pts',(-26.0718209580446,-81.4026693703699,
84.3598599506523));
#179961=CARTESIAN_POINT('Ctrl Pts',(-26.0604409945474,-81.841759782,84.1024337334988));
#179962=CARTESIAN_POINT('Ctrl Pts',(-26.0540874597251,-82.0786814708573,
83.9532153401487));
#179963=CARTESIAN_POINT('Ctrl Pts',(-26.0326197025067,-82.8583908629171,
83.426684350656));
#179964=CARTESIAN_POINT('Ctrl Pts',(-26.0173630094784,-83.3783347810282,
83.0154683355479));
#179965=CARTESIAN_POINT('Ctrl Pts',(-25.9978843357506,-84.0264784016952,
82.4162387348755));
#179966=CARTESIAN_POINT('Ctrl Pts',(-25.9930878128077,-84.1849799764002,
82.2618823059327));
#179967=CARTESIAN_POINT('Ctrl Pts',(-25.9825809313068,-84.5285903864206,
81.9094303283484));
#179968=CARTESIAN_POINT('Ctrl Pts',(-25.9769052402276,-84.7113090086692,
81.7097666897259));
#179969=CARTESIAN_POINT('Ctrl Pts',(-25.961608050232,-85.1874381789504,
81.155737120242));
#179970=CARTESIAN_POINT('Ctrl Pts',(-25.952000205556,-85.4687383554471,
80.7909734609118));
#179971=CARTESIAN_POINT('Ctrl Pts',(-25.9358149717999,-85.8922432586057,
80.1779994751828));
#179972=CARTESIAN_POINT('Ctrl Pts',(-25.9294938723795,-86.0466684166363,
79.9382093144296));
#179973=CARTESIAN_POINT('Ctrl Pts',(-25.9143737003665,-86.393063506594,
79.3600233212961));
#179974=CARTESIAN_POINT('Ctrl Pts',(-25.905510480436,-86.5782227926926,
79.0175079635106));
#179975=CARTESIAN_POINT('Ctrl Pts',(-25.8852182883946,-86.9668909989723,
78.2153442863922));
#179976=CARTESIAN_POINT('Ctrl Pts',(-25.8737960710766,-87.1600185044385,
77.7506301255387));
#179977=CARTESIAN_POINT('Ctrl Pts',(-25.8573459921238,-87.4051241865287,
77.0475922525296));
#179978=CARTESIAN_POINT('Ctrl Pts',(-25.8520764705073,-87.4783803834003,
76.8167470193745));
#179979=CARTESIAN_POINT('Ctrl Pts',(-25.8392195879066,-87.6438771631219,
76.2385212852944));
#179980=CARTESIAN_POINT('Ctrl Pts',(-25.8317245562172,-87.7281208555165,
75.8893932446823));
#179981=CARTESIAN_POINT('Ctrl Pts',(-25.8169812586108,-87.8643090925225,
75.2015789058741));
#179982=CARTESIAN_POINT('Ctrl Pts',(-25.8097174915849,-87.9175609186128,
74.8631684568653));
#179983=CARTESIAN_POINT('Ctrl Pts',(-25.7937813406749,-88.0030548038068,
74.1362254915934));
#179984=CARTESIAN_POINT('Ctrl Pts',(-25.7851028224779,-88.0313761686669,
73.7472133444228));
#179985=CARTESIAN_POINT('Ctrl Pts',(-25.7614798027027,-88.0612328413822,
72.6969835515868));
#179986=CARTESIAN_POINT('Ctrl Pts',(-25.7463802248193,-88.0303757281828,
72.0347225112334));
#179987=CARTESIAN_POINT('Ctrl Pts',(-25.7241993780915,-87.9089029806346,
71.0492587936999));
#179988=CARTESIAN_POINT('Ctrl Pts',(-25.7168688288055,-87.8556904339266,
70.7214147466801));
#179989=CARTESIAN_POINT('Ctrl Pts',(-25.7043057448399,-87.7404526520802,
70.152288399804));
#179990=CARTESIAN_POINT('Ctrl Pts',(-25.6990302602599,-87.6840409946244,
69.9103264370149));
#179991=CARTESIAN_POINT('Ctrl Pts',(-25.6886812995691,-87.5591558926574,
69.4368652277445));
#179992=CARTESIAN_POINT('Ctrl Pts',(-25.6836015556126,-87.4910407607913,
69.2051900647473));
#179993=CARTESIAN_POINT('Ctrl Pts',(-25.6710187955589,-87.3084196999825,
68.6423027329678));
#179994=CARTESIAN_POINT('Ctrl Pts',(-25.6634241156324,-87.1868554521697,
68.3133832130026));
#179995=CARTESIAN_POINT('Ctrl Pts',(-25.6469322102791,-86.8989917421115,
67.6208152365593));
#179996=CARTESIAN_POINT('Ctrl Pts',(-25.6380101285661,-86.7287897905199,
67.2587491966665));
#179997=CARTESIAN_POINT('Ctrl Pts',(-25.6094817159753,-86.1360404434086,
66.1334748648337));
#179998=CARTESIAN_POINT('Ctrl Pts',(-25.5897208421621,-85.6529542244707,
65.4019430271132));
#179999=CARTESIAN_POINT('Ctrl Pts',(-25.5633037283315,-84.8859514128838,
64.4631656614516));
#180000=CARTESIAN_POINT('Ctrl Pts',(-25.5560718741698,-84.661096504945,
64.2093152050967));
#180001=CARTESIAN_POINT('Ctrl Pts',(-25.5376322776274,-84.0614744011126,
63.5839901608553));
#180002=CARTESIAN_POINT('Ctrl Pts',(-25.5262669865481,-83.6735836414418,
63.2260754919771));
#180003=CARTESIAN_POINT('Ctrl Pts',(-25.5015769616827,-82.8034571212361,
62.5149304690227));
#180004=CARTESIAN_POINT('Ctrl Pts',(-25.4882596372729,-82.3154604851025,
62.1686024899682));
#180005=CARTESIAN_POINT('Ctrl Pts',(-25.4563913029029,-81.0970264860667,
61.4226454677198));
#180006=CARTESIAN_POINT('Ctrl Pts',(-25.4378456322442,-80.3465179806126,
61.0554992253828));
#180007=CARTESIAN_POINT('Ctrl Pts',(-25.4108569342881,-79.1794003752194,
60.6192454761137));
#180008=CARTESIAN_POINT('Ctrl Pts',(-25.4020110591221,-78.7848331540593,
60.4933124162824));
#180009=CARTESIAN_POINT('Ctrl Pts',(-25.3752278172481,-77.5928758295803,
60.1745015950223));
#180010=CARTESIAN_POINT('Ctrl Pts',(-25.3571272366448,-76.7800838228553,
60.0374753873656));
#180011=CARTESIAN_POINT('Ctrl Pts',(-25.3188691787239,-75.0556604521194,
59.909545036559));
#180012=CARTESIAN_POINT('Ctrl Pts',(-25.2986976871102,-74.142358408256,
59.9358960981425));
#180013=CARTESIAN_POINT('Ctrl Pts',(-25.2583479842648,-72.317055915739,
60.1832535945134));
#180014=CARTESIAN_POINT('Ctrl Pts',(-25.238105754833,-71.4094419108868,
60.4097518282593));
#180015=CARTESIAN_POINT('Ctrl Pts',(-25.2177843835793,-70.5373207047723,
60.7277886365121));
#180016=CARTESIAN_POINT('',(-25.21690938235,-70.5367618819012,60.7262027183532));
#180017=CARTESIAN_POINT('Ctrl Pts',(-29.4261514861327,-77.757911767464,
85.74414017529));
#180018=CARTESIAN_POINT('Ctrl Pts',(-29.3779431821827,-79.904349121914,
85.28004229623));
#180019=CARTESIAN_POINT('Ctrl Pts',(-29.2815265742827,-83.95514758824,83.24564128978));
#180020=CARTESIAN_POINT('Ctrl Pts',(-29.1369016624246,-87.79923337781,77.634595795182));
#180021=CARTESIAN_POINT('Ctrl Pts',(-28.9922767505727,-88.44943474654,70.864604569967));
#180022=CARTESIAN_POINT('Ctrl Pts',(-28.8476518387227,-85.74425521307,64.624573520997));
#180023=CARTESIAN_POINT('Ctrl Pts',(-28.7030269268629,-80.358422966095,
60.47138590026));
#180024=CARTESIAN_POINT('Ctrl Pts',(-28.5584020150127,-73.635715047619,
59.44121987509));
#180025=CARTESIAN_POINT('Ctrl Pts',(-28.4137771031546,-67.253383129327,
61.79109721394));
#180026=CARTESIAN_POINT('Ctrl Pts',(-28.2691521913028,-62.80377526215,66.934740200613));
#180027=CARTESIAN_POINT('Ctrl Pts',(-28.1245272794527,-61.39703449716,73.5888484027236));
#180028=CARTESIAN_POINT('Ctrl Pts',(-27.9799023675929,-63.38413245482,80.093271282679));
#180029=CARTESIAN_POINT('Ctrl Pts',(-27.8352774557427,-68.269302909975,
84.82520375033));
#180030=CARTESIAN_POINT('Ctrl Pts',(-27.6906525438927,-74.8337322064467,
86.60406386368));
#180031=CARTESIAN_POINT('Ctrl Pts',(-27.5460276320329,-81.439644079033,
84.98603926299));
#180032=CARTESIAN_POINT('Ctrl Pts',(-27.4014027201827,-86.43891267502,80.374815045269));
#180033=CARTESIAN_POINT('Ctrl Pts',(-27.2567778083246,-88.58425768156,73.9208573383313));
#180034=CARTESIAN_POINT('Ctrl Pts',(-27.1121528964728,-87.34043148427,67.234380562697));
#180035=CARTESIAN_POINT('Ctrl Pts',(-26.9675279846227,-83.017759463383,
61.98361091626));
#180036=CARTESIAN_POINT('Ctrl Pts',(-26.8229030727646,-76.694716120822,
59.47857635201));
#180037=CARTESIAN_POINT('Ctrl Pts',(-26.6782781609127,-69.94885371734,60.34426435248));
#180038=CARTESIAN_POINT('Ctrl Pts',(-26.5336532490595,-64.46321472334,64.36469220339));
#180039=CARTESIAN_POINT('Ctrl Pts',(-26.3890283372062,-61.60642524515,70.536793074933));
#180040=CARTESIAN_POINT('Ctrl Pts',(-26.2444034253522,-62.09123300285,77.320673726326));
#180041=CARTESIAN_POINT('Ctrl Pts',(-26.0997785134991,-65.796682053056,
83.02380642958));
#180042=CARTESIAN_POINT('Ctrl Pts',(-25.9551536016452,-71.798290489993,
86.22330197028));
#180043=CARTESIAN_POINT('Ctrl Pts',(-25.8105286897922,-78.59870145323,86.12091018816));
#180044=CARTESIAN_POINT('Ctrl Pts',(-25.665903777939,-84.50126382125,82.742176443924));
#180045=CARTESIAN_POINT('Ctrl Pts',(-25.5212788660852,-88.03332919063,76.930072003796));
#180046=CARTESIAN_POINT('Ctrl Pts',(-25.3766539542322,-88.31368479424,70.134664941592));
#180047=CARTESIAN_POINT('Ctrl Pts',(-25.2320290423791,-85.27234197776,64.051391343194));
#180048=CARTESIAN_POINT('Ctrl Pts',(-25.0874041305261,-79.668249953127,
60.1978610671));
#180049=CARTESIAN_POINT('Ctrl Pts',(-24.942779218673,-72.899002749005,59.53595519057));
#180050=CARTESIAN_POINT('Ctrl Pts',(-24.846362610771,-68.736775097357,61.33139849116));
#180051=CARTESIAN_POINT('Ctrl Pts',(-24.79815430682,-67.001564902287,62.6773649606));
#180052=CARTESIAN_POINT('Ctrl Pts',(-29.5486931499337,-77.757911767464,
85.74414017529));
#180053=CARTESIAN_POINT('Ctrl Pts',(-29.5004848459837,-79.904349121914,
85.28004229623));
#180054=CARTESIAN_POINT('Ctrl Pts',(-29.4040682380836,-83.95514758824,83.24564128978));
#180055=CARTESIAN_POINT('Ctrl Pts',(-29.2594433262332,-87.79923337781,77.634595795182));
#180056=CARTESIAN_POINT('Ctrl Pts',(-29.1148184143737,-88.44943474654,70.864604569967));
#180057=CARTESIAN_POINT('Ctrl Pts',(-28.9701935025236,-85.74425521307,64.624573520997));
#180058=CARTESIAN_POINT('Ctrl Pts',(-28.8255685906649,-80.358422966095,
60.47138590026));
#180059=CARTESIAN_POINT('Ctrl Pts',(-28.6809436788136,-73.635715047619,
59.44121987509));
#180060=CARTESIAN_POINT('Ctrl Pts',(-28.5363187669632,-67.253383129327,
61.79109721394));
#180061=CARTESIAN_POINT('Ctrl Pts',(-28.3916938551037,-62.80377526215,66.934740200613));
#180062=CARTESIAN_POINT('Ctrl Pts',(-28.2470689432536,-61.39703449716,73.5888484027236));
#180063=CARTESIAN_POINT('Ctrl Pts',(-28.1024440313949,-63.38413245482,80.093271282679));
#180064=CARTESIAN_POINT('Ctrl Pts',(-27.9578191195436,-68.269302909975,
84.82520375033));
#180065=CARTESIAN_POINT('Ctrl Pts',(-27.8131942076936,-74.8337322064467,
86.60406386368));
#180066=CARTESIAN_POINT('Ctrl Pts',(-27.6685692958349,-81.439644079033,
84.98603926299));
#180067=CARTESIAN_POINT('Ctrl Pts',(-27.5239443839836,-86.43891267502,80.374815045269));
#180068=CARTESIAN_POINT('Ctrl Pts',(-27.3793194721332,-88.58425768156,73.9208573383313));
#180069=CARTESIAN_POINT('Ctrl Pts',(-27.2346945602737,-87.34043148427,67.234380562697));
#180070=CARTESIAN_POINT('Ctrl Pts',(-27.0900696484237,-83.017759463383,
61.98361091626));
#180071=CARTESIAN_POINT('Ctrl Pts',(-26.9454447365732,-76.694716120822,
59.47857635201));
#180072=CARTESIAN_POINT('Ctrl Pts',(-26.8008198247137,-69.94885371734,60.34426435248));
#180073=CARTESIAN_POINT('Ctrl Pts',(-26.6561949128635,-64.46321472334,64.36469220339));
#180074=CARTESIAN_POINT('Ctrl Pts',(-26.5115700010092,-61.60642524515,70.536793074933));
#180075=CARTESIAN_POINT('Ctrl Pts',(-26.3669450891548,-62.09123300285,77.320673726326));
#180076=CARTESIAN_POINT('Ctrl Pts',(-26.2223201773017,-65.796682053056,
83.02380642958));
#180077=CARTESIAN_POINT('Ctrl Pts',(-26.0776952654478,-71.798290489993,
86.22330197028));
#180078=CARTESIAN_POINT('Ctrl Pts',(-25.9330703535948,-78.59870145323,86.12091018816));
#180079=CARTESIAN_POINT('Ctrl Pts',(-25.7884454417409,-84.50126382125,82.742176443924));
#180080=CARTESIAN_POINT('Ctrl Pts',(-25.6438205298878,-88.03332919063,76.930072003796));
#180081=CARTESIAN_POINT('Ctrl Pts',(-25.4991956180348,-88.31368479424,70.134664941592));
#180082=CARTESIAN_POINT('Ctrl Pts',(-25.3545707061817,-85.27234197776,64.051391343194));
#180083=CARTESIAN_POINT('Ctrl Pts',(-25.2099457943287,-79.668249953127,
60.1978610671));
#180084=CARTESIAN_POINT('Ctrl Pts',(-25.0653208824749,-72.899002749005,
59.53595519057));
#180085=CARTESIAN_POINT('Ctrl Pts',(-24.9689042745729,-68.736775097357,
61.33139849116));
#180086=CARTESIAN_POINT('Ctrl Pts',(-24.9206959706219,-67.001564902287,
62.6773649606));
#180087=CARTESIAN_POINT('Ctrl Pts',(-29.6712348137352,-77.757911767464,
85.74414017529));
#180088=CARTESIAN_POINT('Ctrl Pts',(-29.6230265097852,-79.904349121914,
85.28004229623));
#180089=CARTESIAN_POINT('Ctrl Pts',(-29.5266099018845,-83.95514758824,83.24564128978));
#180090=CARTESIAN_POINT('Ctrl Pts',(-29.3819849900345,-87.79923337781,77.634595795182));
#180091=CARTESIAN_POINT('Ctrl Pts',(-29.2373600781752,-88.44943474654,70.864604569967));
#180092=CARTESIAN_POINT('Ctrl Pts',(-29.0927351663245,-85.74425521307,64.624573520997));
#180093=CARTESIAN_POINT('Ctrl Pts',(-28.9481102544736,-80.358422966095,
60.47138590026));
#180094=CARTESIAN_POINT('Ctrl Pts',(-28.8034853426145,-73.635715047619,
59.44121987509));
#180095=CARTESIAN_POINT('Ctrl Pts',(-28.6588604307645,-67.253383129327,
61.79109721394));
#180096=CARTESIAN_POINT('Ctrl Pts',(-28.5142355189052,-62.80377526215,66.934740200613));
#180097=CARTESIAN_POINT('Ctrl Pts',(-28.3696106070545,-61.39703449716,73.5888484027236));
#180098=CARTESIAN_POINT('Ctrl Pts',(-28.2249856952036,-63.38413245482,80.093271282679));
#180099=CARTESIAN_POINT('Ctrl Pts',(-28.0803607833445,-68.269302909975,
84.82520375033));
#180100=CARTESIAN_POINT('Ctrl Pts',(-27.9357358714945,-74.8337322064467,
86.60406386368));
#180101=CARTESIAN_POINT('Ctrl Pts',(-27.7911109596436,-81.439644079033,
84.98603926299));
#180102=CARTESIAN_POINT('Ctrl Pts',(-27.6464860477845,-86.43891267502,80.374815045269));
#180103=CARTESIAN_POINT('Ctrl Pts',(-27.5018611359345,-88.58425768156,73.9208573383313));
#180104=CARTESIAN_POINT('Ctrl Pts',(-27.3572362240752,-87.34043148427,67.234380562697));
#180105=CARTESIAN_POINT('Ctrl Pts',(-27.2126113122245,-83.017759463383,
61.98361091626));
#180106=CARTESIAN_POINT('Ctrl Pts',(-27.0679864003745,-76.694716120822,
59.47857635201));
#180107=CARTESIAN_POINT('Ctrl Pts',(-26.9233614885152,-69.94885371734,60.34426435248));
#180108=CARTESIAN_POINT('Ctrl Pts',(-26.7787365766645,-64.46321472334,64.36469220339));
#180109=CARTESIAN_POINT('Ctrl Pts',(-26.6341116648141,-61.60642524515,70.536793074933));
#180110=CARTESIAN_POINT('Ctrl Pts',(-26.4894867529572,-62.09123300285,77.320673726326));
#180111=CARTESIAN_POINT('Ctrl Pts',(-26.3448618411036,-65.796682053056,
83.02380642958));
#180112=CARTESIAN_POINT('Ctrl Pts',(-26.2002369292505,-71.798290489993,
86.22330197028));
#180113=CARTESIAN_POINT('Ctrl Pts',(-26.0556120173974,-78.59870145323,86.12091018816));
#180114=CARTESIAN_POINT('Ctrl Pts',(-25.9109871055435,-84.50126382125,82.742176443924));
#180115=CARTESIAN_POINT('Ctrl Pts',(-25.7663621936905,-88.03332919063,76.930072003796));
#180116=CARTESIAN_POINT('Ctrl Pts',(-25.6217372818374,-88.31368479424,70.134664941592));
#180117=CARTESIAN_POINT('Ctrl Pts',(-25.4771123699836,-85.27234197776,64.051391343194));
#180118=CARTESIAN_POINT('Ctrl Pts',(-25.3324874581306,-79.668249953127,
60.1978610671));
#180119=CARTESIAN_POINT('Ctrl Pts',(-25.1878625462775,-72.899002749005,
59.53595519057));
#180120=CARTESIAN_POINT('Ctrl Pts',(-25.0914459383755,-68.736775097357,
61.33139849116));
#180121=CARTESIAN_POINT('Ctrl Pts',(-25.0432376344245,-67.001564902287,
62.6773649606));
#180122=CARTESIAN_POINT('Ctrl Pts',(-29.793776477544,-77.757911767464,85.74414017529));
#180123=CARTESIAN_POINT('Ctrl Pts',(-29.745568173594,-79.904349121914,85.28004229623));
#180124=CARTESIAN_POINT('Ctrl Pts',(-29.6491515656854,-83.95514758824,83.24564128978));
#180125=CARTESIAN_POINT('Ctrl Pts',(-29.5045266538354,-87.79923337781,77.634595795182));
#180126=CARTESIAN_POINT('Ctrl Pts',(-29.359901741984,-88.44943474654,70.864604569967));
#180127=CARTESIAN_POINT('Ctrl Pts',(-29.2152768301254,-85.74425521307,64.624573520997));
#180128=CARTESIAN_POINT('Ctrl Pts',(-29.0706519182754,-80.358422966095,
60.47138590026));
#180129=CARTESIAN_POINT('Ctrl Pts',(-28.9260270064154,-73.635715047619,
59.44121987509));
#180130=CARTESIAN_POINT('Ctrl Pts',(-28.7814020945654,-67.253383129327,
61.79109721394));
#180131=CARTESIAN_POINT('Ctrl Pts',(-28.636777182714,-62.80377526215,66.934740200613));
#180132=CARTESIAN_POINT('Ctrl Pts',(-28.4921522708554,-61.39703449716,73.5888484027236));
#180133=CARTESIAN_POINT('Ctrl Pts',(-28.3475273590054,-63.38413245482,80.093271282679));
#180134=CARTESIAN_POINT('Ctrl Pts',(-28.2029024471454,-68.269302909975,
84.82520375033));
#180135=CARTESIAN_POINT('Ctrl Pts',(-28.0582775352954,-74.8337322064467,
86.60406386368));
#180136=CARTESIAN_POINT('Ctrl Pts',(-27.9136526234454,-81.439644079033,
84.98603926299));
#180137=CARTESIAN_POINT('Ctrl Pts',(-27.7690277115854,-86.43891267502,80.374815045269));
#180138=CARTESIAN_POINT('Ctrl Pts',(-27.6244027997354,-88.58425768156,73.9208573383313));
#180139=CARTESIAN_POINT('Ctrl Pts',(-27.479777887884,-87.34043148427,67.234380562697));
#180140=CARTESIAN_POINT('Ctrl Pts',(-27.3351529760254,-83.017759463383,
61.98361091626));
#180141=CARTESIAN_POINT('Ctrl Pts',(-27.1905280641754,-76.694716120822,
59.47857635201));
#180142=CARTESIAN_POINT('Ctrl Pts',(-27.045903152324,-69.94885371734,60.34426435248));
#180143=CARTESIAN_POINT('Ctrl Pts',(-26.9012782404654,-64.46321472334,64.36469220339));
#180144=CARTESIAN_POINT('Ctrl Pts',(-26.7566533286154,-61.60642524515,70.536793074933));
#180145=CARTESIAN_POINT('Ctrl Pts',(-26.6120284167559,-62.09123300285,77.320673726326));
#180146=CARTESIAN_POINT('Ctrl Pts',(-26.4674035049062,-65.796682053056,
83.02380642958));
#180147=CARTESIAN_POINT('Ctrl Pts',(-26.3227785930532,-71.798290489993,
86.22330197028));
#180148=CARTESIAN_POINT('Ctrl Pts',(-26.1781536811993,-78.59870145323,86.12091018816));
#180149=CARTESIAN_POINT('Ctrl Pts',(-26.0335287693461,-84.50126382125,82.742176443924));
#180150=CARTESIAN_POINT('Ctrl Pts',(-25.8889038574932,-88.03332919063,76.930072003796));
#180151=CARTESIAN_POINT('Ctrl Pts',(-25.7442789456393,-88.31368479424,70.134664941592));
#180152=CARTESIAN_POINT('Ctrl Pts',(-25.5996540337862,-85.27234197776,64.051391343194));
#180153=CARTESIAN_POINT('Ctrl Pts',(-25.4550291219332,-79.668249953127,
60.1978610671));
#180154=CARTESIAN_POINT('Ctrl Pts',(-25.3104042100802,-72.899002749005,
59.53595519057));
#180155=CARTESIAN_POINT('Ctrl Pts',(-25.2139876021782,-68.736775097357,
61.33139849116));
#180156=CARTESIAN_POINT('Ctrl Pts',(-25.1657792982272,-67.001564902287,
62.6773649606));
#180157=CARTESIAN_POINT('Ctrl Pts',(-29.3655838523953,-81.6013626746983,
84.2438270474911));
#180158=CARTESIAN_POINT('Ctrl Pts',(-29.3303036656744,-82.9881381538602,
83.4317063126598));
#180159=CARTESIAN_POINT('Ctrl Pts',(-29.295627364516,-84.2015222616406,
82.3803230252726));
#180160=CARTESIAN_POINT('Ctrl Pts',(-29.2347381075074,-85.9289061095604,
80.2099621171966));
#180161=CARTESIAN_POINT('Ctrl Pts',(-29.1967714573928,-86.9123357997735,
78.737499184749));
#180162=CARTESIAN_POINT('Ctrl Pts',(-29.1127653603425,-87.9905194137987,
75.0668637575484));
#180163=CARTESIAN_POINT('Ctrl Pts',(-29.075894631943,-88.150447003745,73.3629071254178));
#180164=CARTESIAN_POINT('Ctrl Pts',(-28.9922442448894,-87.7751516038179,
69.5720079624225));
#180165=CARTESIAN_POINT('Ctrl Pts',(-28.9538064145164,-87.08512602708,67.9181509720035));
#180166=CARTESIAN_POINT('Ctrl Pts',(-28.8854503569788,-85.6164657565867,
65.1722907800833));
#180167=CARTESIAN_POINT('Ctrl Pts',(-28.8482263560423,-84.4707456685075,
63.8773740095143));
#180168=CARTESIAN_POINT('Ctrl Pts',(-28.7869286879839,-82.3077021213379,
62.1109491954591));
#180169=CARTESIAN_POINT('Ctrl Pts',(-28.749043597868,-80.8425902128494,
61.1249202595487));
#180170=CARTESIAN_POINT('Ctrl Pts',(-28.6656746731545,-77.2087891219336,
60.0229950603655));
#180171=CARTESIAN_POINT('Ctrl Pts',(-28.6291541528475,-75.523734318193,
59.8442380189927));
#180172=CARTESIAN_POINT('Ctrl Pts',(-28.5552353989383,-72.170375446941,
60.1356096181979));
#180173=CARTESIAN_POINT('Ctrl Pts',(-28.5179385729897,-70.5085301046633,
60.622769542381));
#180174=CARTESIAN_POINT('Ctrl Pts',(-28.4325907303431,-67.0540816724184,
62.4060056730254));
#180175=CARTESIAN_POINT('Ctrl Pts',(-28.3942903930223,-65.7896559531696,
63.6694196806761));
#180176=CARTESIAN_POINT('Ctrl Pts',(-28.3368489710222,-64.1046749841286,
65.6718124865969));
#180177=CARTESIAN_POINT('Ctrl Pts',(-28.2993959861414,-63.1656332196875,
67.1384103391823));
#180178=CARTESIAN_POINT('Ctrl Pts',(-28.2228502956743,-62.1131264080113,
70.4626573346813));
#180179=CARTESIAN_POINT('Ctrl Pts',(-28.1861287854086,-61.8461477642845,
72.1469332660689));
#180180=CARTESIAN_POINT('Ctrl Pts',(-28.1085461465717,-62.1183832603,75.6693497096584));
#180181=CARTESIAN_POINT('Ctrl Pts',(-28.071489187918,-62.5795360968161,
77.3267817400747));
#180182=CARTESIAN_POINT('Ctrl Pts',(-27.9868394695533,-64.3034330597131,
80.7751238150644));
#180183=CARTESIAN_POINT('Ctrl Pts',(-27.9484187558418,-65.548506983732,
82.0646263543977));
#180184=CARTESIAN_POINT('Ctrl Pts',(-27.8840027503118,-67.7671789913901,
83.9854448061143));
#180185=CARTESIAN_POINT('Ctrl Pts',(-27.8469128057308,-69.2644434892098,
84.8353927582126));
#180186=CARTESIAN_POINT('Ctrl Pts',(-27.7827496034337,-72.0399537191075,
85.7525454179823));
#180187=CARTESIAN_POINT('Ctrl Pts',(-27.7448787069659,-73.7589969853065,
86.1552553504063));
#180188=CARTESIAN_POINT('Ctrl Pts',(-27.6613031356659,-77.5561960000081,
85.8925693173151));
#180189=CARTESIAN_POINT('Ctrl Pts',(-27.6245645194847,-79.2040488916052,
85.454539118987));
#180190=CARTESIAN_POINT('Ctrl Pts',(-27.545723918875,-82.4335893984305,
83.8861011614419));
#180191=CARTESIAN_POINT('Ctrl Pts',(-27.5081701457295,-83.7695689881318,
82.7623462776217));
#180192=CARTESIAN_POINT('Ctrl Pts',(-27.431506954629,-86.0909832894995,
80.1533697833587));
#180193=CARTESIAN_POINT('Ctrl Pts',(-27.3938450433658,-86.871569728093,
78.585244494142));
#180194=CARTESIAN_POINT('Ctrl Pts',(-27.3365640377179,-87.7227218052663,
76.1182439307786));
#180195=CARTESIAN_POINT('Ctrl Pts',(-27.2985997691106,-88.1554259539642,
74.4007921117372));
#180196=CARTESIAN_POINT('Ctrl Pts',(-27.2144471677441,-87.9283326232303,
70.5744157048114));
#180197=CARTESIAN_POINT('Ctrl Pts',(-27.1780151180434,-87.5152757592269,
68.9354836726551));
#180198=CARTESIAN_POINT('Ctrl Pts',(-27.1051166195486,-86.1018611225955,
65.9319091457066));
#180199=CARTESIAN_POINT('Ctrl Pts',(-27.0686837698037,-85.1030263512263,
64.5683559877304));
#180200=CARTESIAN_POINT('Ctrl Pts',(-26.9839443790261,-82.2803880750339,
61.9357859485765));
#180201=CARTESIAN_POINT('Ctrl Pts',(-26.9459015379113,-80.6723964065564,
61.1819992045571));
#180202=CARTESIAN_POINT('Ctrl Pts',(-26.8876102860954,-78.1864303986462,
60.2477452459039));
#180203=CARTESIAN_POINT('Ctrl Pts',(-26.8502010969373,-76.4872594038116,
59.8797505089315));
#180204=CARTESIAN_POINT('Ctrl Pts',(-26.7761028839489,-73.1139235187851,
59.9992914624847));
#180205=CARTESIAN_POINT('Ctrl Pts',(-26.7384047115212,-71.3858814275703,
60.2955114455625));
#180206=CARTESIAN_POINT('Ctrl Pts',(-26.6585341496444,-68.0757772917095,
61.8029934063736));
#180207=CARTESIAN_POINT('Ctrl Pts',(-26.6217434954712,-66.685638534737,
62.7946497723639));
#180208=CARTESIAN_POINT('Ctrl Pts',(-26.5367444780904,-64.0190722193934,
65.6007532047943));
#180209=CARTESIAN_POINT('Ctrl Pts',(-26.4986415165783,-63.2510209027794,
67.2052974950793));
#180210=CARTESIAN_POINT('Ctrl Pts',(-26.4362248200088,-62.2166753702092,
69.854018890858));
#180211=CARTESIAN_POINT('Ctrl Pts',(-26.399137480781,-61.9174125243928,
71.5493285777501));
#180212=CARTESIAN_POINT('Ctrl Pts',(-26.3345682468581,-61.9819953219415,
74.4902614964466));
#180213=CARTESIAN_POINT('Ctrl Pts',(-26.2962027710617,-62.183439931008,
76.2685907288007));
#180214=CARTESIAN_POINT('Ctrl Pts',(-26.2116136533861,-63.739688531473,
79.7928374527053));
#180215=CARTESIAN_POINT('Ctrl Pts',(-26.1745142485159,-64.7236347634373,
81.2065457467117));
#180216=CARTESIAN_POINT('Ctrl Pts',(-26.0976814723829,-67.24032118938,83.6370669645294));
#180217=CARTESIAN_POINT('Ctrl Pts',(-26.061001678293,-68.699461980102,84.5148158415022));
#180218=CARTESIAN_POINT('Ctrl Pts',(-25.9817789563583,-72.0440939057269,
85.8700472606708));
#180219=CARTESIAN_POINT('Ctrl Pts',(-25.9440135851621,-73.7936835266116,
86.0461011698092));
#180220=CARTESIAN_POINT('Ctrl Pts',(-25.8883468613303,-76.3297703438795,
86.026800080011));
#180221=CARTESIAN_POINT('Ctrl Pts',(-25.8501294132487,-78.1034545947031,
85.8493490383469));
#180222=CARTESIAN_POINT('Ctrl Pts',(-25.7675740621284,-81.5634937701812,
84.3765890039492));
#180223=CARTESIAN_POINT('Ctrl Pts',(-25.7302992652139,-83.0209293484797,
83.4417113170998));
#180224=CARTESIAN_POINT('Ctrl Pts',(-25.6539646250139,-85.4607500576467,
80.9658198961807));
#180225=CARTESIAN_POINT('Ctrl Pts',(-25.6173876023457,-86.3989869481063,
79.5514735758963));
#180226=CARTESIAN_POINT('Ctrl Pts',(-25.53394245796,-87.8666834060939,76.0457160962318));
#180227=CARTESIAN_POINT('Ctrl Pts',(-25.4960524688697,-88.0394369527268,
74.2878474727088));
#180228=CARTESIAN_POINT('Ctrl Pts',(-25.4316021534887,-88.0588502759257,
71.3516283557702));
#180229=CARTESIAN_POINT('Ctrl Pts',(-25.3944251791231,-87.7342041208073,
69.6567021743647));
#180230=CARTESIAN_POINT('Ctrl Pts',(-25.3304167651469,-86.6305562570029,
66.9576863201386));
#180231=CARTESIAN_POINT('Ctrl Pts',(-25.2918432869613,-85.8084429463678,
65.3563934455804));
#180232=CARTESIAN_POINT('Ctrl Pts',(-25.2071469265164,-83.0931608647546,
62.6169175361423));
#180233=CARTESIAN_POINT('Ctrl Pts',(-25.170226450455,-81.6763364745364,
61.6526283543061));
#180234=CARTESIAN_POINT('Ctrl Pts',(-25.0872961958142,-78.2051085262274,
60.1648056900112));
#180235=CARTESIAN_POINT('Ctrl Pts',(-25.0495042431519,-76.455634995068,
59.9662747528024));
#180236=CARTESIAN_POINT('Ctrl Pts',(-24.9874702782534,-73.6301866430724,
59.9123510791511));
#180237=CARTESIAN_POINT('Ctrl Pts',(-24.9527649126985,-72.0454497036876,
60.1778193699471));
#180238=CARTESIAN_POINT('Ctrl Pts',(-24.9175248385795,-70.5373262934946,
60.7277865984718));
#180239=CARTESIAN_POINT('Ctrl Pts',(-24.5840827087049,-75.4257087102522,
60.79818693484));
#180240=CARTESIAN_POINT('Ctrl Pts',(-24.5542910420379,-74.1579666637678,
60.75391640706));
#180241=CARTESIAN_POINT('Ctrl Pts',(-24.4947077087039,-71.60879259167,61.06410883866));
#180242=CARTESIAN_POINT('Ctrl Pts',(-24.4053327087039,-68.112244415052,
62.68064695513));
#180243=CARTESIAN_POINT('Ctrl Pts',(-24.3159577087039,-65.280711439107,
65.292377040265));
#180244=CARTESIAN_POINT('Ctrl Pts',(-24.2265827087039,-63.38749595989,68.647152239787));
#180245=CARTESIAN_POINT('Ctrl Pts',(-24.1372077087039,-62.61539180617,72.4210925622802));
#180246=CARTESIAN_POINT('Ctrl Pts',(-24.0478327087039,-63.0389358374,76.249849747832));
#180247=CARTESIAN_POINT('Ctrl Pts',(-23.9584577087039,-64.61723898556,79.7637835434));
#180248=CARTESIAN_POINT('Ctrl Pts',(-23.8690827087039,-67.197926562624,
82.623647685499));
#180249=CARTESIAN_POINT('Ctrl Pts',(-23.7797077087039,-70.531850936755,
84.55334187238));
#180250=CARTESIAN_POINT('Ctrl Pts',(-23.6903327087039,-74.297144509849,
85.36656733984));
#180251=CARTESIAN_POINT('Ctrl Pts',(-23.6009577087039,-78.130293970206,
84.98481273641));
#180252=CARTESIAN_POINT('Ctrl Pts',(-23.5115827087039,-81.661234976842,
83.44493385557));
#180253=CARTESIAN_POINT('Ctrl Pts',(-23.4222077087039,-84.549079348228,
80.895595461536));
#180254=CARTESIAN_POINT('Ctrl Pts',(-23.3328327087039,-86.51502547987,77.582918723914));
#180255=CARTESIAN_POINT('Ctrl Pts',(-23.2434577087039,-87.36927473133,73.8267199037071));
#180256=CARTESIAN_POINT('Ctrl Pts',(-23.1540827087039,-87.02935518539,69.989634282714));
#180257=CARTESIAN_POINT('Ctrl Pts',(-23.0647077087039,-85.52808374721,66.442106209615));
#180258=CARTESIAN_POINT('Ctrl Pts',(-22.9753327087039,-83.01039789668,63.5266252341));
#180259=CARTESIAN_POINT('Ctrl Pts',(-22.8859577087039,-79.719362967031,
61.52466108548));
#180260=CARTESIAN_POINT('Ctrl Pts',(-22.7965827087039,-75.9727058508626,
60.62948969719));
#180261=CARTESIAN_POINT('Ctrl Pts',(-22.7072077087039,-72.132140643769,
60.92753373859));
#180262=CARTESIAN_POINT('Ctrl Pts',(-22.6178327087039,-68.568447624649,
62.39001909784));
#180263=CARTESIAN_POINT('Ctrl Pts',(-22.5284577087039,-65.625676958068,
64.875752825426));
#180264=CARTESIAN_POINT('Ctrl Pts',(-22.4390827087039,-63.58793300618,68.144754346856));
#180265=CARTESIAN_POINT('Ctrl Pts',(-22.3497077087039,-62.65194599751,71.881423944257));
#180266=CARTESIAN_POINT('Ctrl Pts',(-22.2603327087039,-62.90807907012,75.725011748597));
#180267=CARTESIAN_POINT('Ctrl Pts',(-22.1709577087039,-64.3316043293,79.304445669906));
#180268=CARTESIAN_POINT('Ctrl Pts',(-22.0815827087039,-66.785090156491,
82.274155867271));
#180269=CARTESIAN_POINT('Ctrl Pts',(-21.9922077087039,-70.031669291213,
84.34743715126));
#180270=CARTESIAN_POINT('Ctrl Pts',(-21.9028327087039,-73.757906743531,
85.32412840723));
#180271=CARTESIAN_POINT('Ctrl Pts',(-21.8134577087039,-77.604059796605,
85.10993678068));
#180272=CARTESIAN_POINT('Ctrl Pts',(-21.7240827087039,-81.198808703261,
83.72554100684));
#180273=CARTESIAN_POINT('Ctrl Pts',(-21.6347077087039,-84.195105065595,
81.304595020325));
#180274=CARTESIAN_POINT('Ctrl Pts',(-21.5453327087049,-86.30367698195,78.080824582763));
#180275=CARTESIAN_POINT('Ctrl Pts',(-21.4559577087049,-87.32095626873,74.365462660522));
#180276=CARTESIAN_POINT('Ctrl Pts',(-21.3665827087049,-87.1487315749,70.517202012466));
#180277=CARTESIAN_POINT('Ctrl Pts',(-21.2772077087049,-85.80363001565,66.907565859634));
#180278=CARTESIAN_POINT('Ctrl Pts',(-21.1878327087049,-83.415511938176,
63.885039861635));
#180279=CARTESIAN_POINT('Ctrl Pts',(-21.0984577087049,-80.214933794219,
61.74142821188));
#180280=CARTESIAN_POINT('Ctrl Pts',(-21.0090827087049,-76.510889492969,
60.68368194036));
#180281=CARTESIAN_POINT('Ctrl Pts',(-20.9197077087049,-72.660979154464,
60.81391920844));
#180282=CARTESIAN_POINT('Ctrl Pts',(-20.8303327087049,-69.036885266062,
62.11956649947));
#180283=CARTESIAN_POINT('Ctrl Pts',(-20.7409577087049,-65.988489282763,
64.474572505729));
#180284=CARTESIAN_POINT('Ctrl Pts',(-20.6515827087049,-63.81009296796,67.651577519286));
#180285=CARTESIAN_POINT('Ctrl Pts',(-20.5622077087049,-62.71200557292,71.343863455311));
#180286=CARTESIAN_POINT('Ctrl Pts',(-20.4728327087049,-62.80023991832,75.194965383434));
#180287=CARTESIAN_POINT('Ctrl Pts',(-20.3834577087049,-64.06627758214,78.833085776478));
#180288=CARTESIAN_POINT('Ctrl Pts',(-20.2940827087049,-66.387891295025,
81.90698901644));
#180289=CARTESIAN_POINT('Ctrl Pts',(-20.2047077087049,-69.540945146354,
84.11991078892));
#180290=CARTESIAN_POINT('Ctrl Pts',(-20.1153327087049,-73.22103337205,85.25820864606));
#180291=CARTESIAN_POINT('Ctrl Pts',(-20.0259577087049,-77.07286864717,85.21198772236));
#180292=CARTESIAN_POINT('Ctrl Pts',(-19.9365827087049,-80.724582644921,
83.98571033155));
#180293=CARTESIAN_POINT('Ctrl Pts',(-19.8472077087049,-83.823627377769,
81.697765160933));
#180294=CARTESIAN_POINT('Ctrl Pts',(-19.7578327087049,-86.0708112925,78.569037653464));
#180295=CARTESIAN_POINT('Ctrl Pts',(-19.6684577087049,-87.24918416519,74.90158503273));
#180296=CARTESIAN_POINT('Ctrl Pts',(-19.5790827087049,-87.24498216486,71.049474737007));
#180297=CARTESIAN_POINT('Ctrl Pts',(-19.4897077087049,-86.05861095495,67.384601665003));
#180298=CARTESIAN_POINT('Ctrl Pts',(-19.4003327087049,-83.804606594842,
64.260784146057));
#180299=CARTESIAN_POINT('Ctrl Pts',(-19.3109577087049,-80.700577622844,
61.97960566264));
#180300=CARTESIAN_POINT('Ctrl Pts',(-19.2215827087049,-77.046197354344,
60.7612973129));
#180301=CARTESIAN_POINT('Ctrl Pts',(-19.1322077087049,-73.194269067977,
60.72348241298));
#180302=CARTESIAN_POINT('Ctrl Pts',(-19.0428327087049,-69.51667797846,61.86979685924));
#180303=CARTESIAN_POINT('Ctrl Pts',(-18.9534577087039,-66.368440815114,
64.089627347503));
#180304=CARTESIAN_POINT('Ctrl Pts',(-18.8938743753709,-64.82521925324,66.1421806368));
#180305=CARTESIAN_POINT('Ctrl Pts',(-18.8640827087039,-64.2296876317,67.262212718386));
#180306=CARTESIAN_POINT('Ctrl Pts',(-24.7409006782679,-75.4362219922699,
60.49712592814));
#180307=CARTESIAN_POINT('Ctrl Pts',(-24.7111090116019,-74.1371718486303,
60.45176209751));
#180308=CARTESIAN_POINT('Ctrl Pts',(-24.6515256782679,-71.52504349515,60.76961502662));
#180309=CARTESIAN_POINT('Ctrl Pts',(-24.5621506782679,-67.942144731418,
62.42607509136));
#180310=CARTESIAN_POINT('Ctrl Pts',(-24.4727756782679,-65.04068435206,65.102304338201));
#180311=CARTESIAN_POINT('Ctrl Pts',(-24.3834006782679,-63.10071411361,68.539928906151));
#180312=CARTESIAN_POINT('Ctrl Pts',(-24.2940256782679,-62.3095421125,72.4070702789702));
#180313=CARTESIAN_POINT('Ctrl Pts',(-24.2046506782679,-62.74354596694,76.330382269486));
#180314=CARTESIAN_POINT('Ctrl Pts',(-24.1152756782679,-64.36082681442,79.931096006583));
#180315=CARTESIAN_POINT('Ctrl Pts',(-24.0259006782679,-67.005246928886,
82.861587217225));
#180316=CARTESIAN_POINT('Ctrl Pts',(-23.9365256782679,-70.421505740455,
84.83893703977));
#180317=CARTESIAN_POINT('Ctrl Pts',(-23.8471506782679,-74.2797868241642,
85.67224588461));
#180318=CARTESIAN_POINT('Ctrl Pts',(-23.7577756782679,-78.207599560894,
85.28106348769));
#180319=CARTESIAN_POINT('Ctrl Pts',(-23.6684006782679,-81.825740518334,
83.70315583141));
#180320=CARTESIAN_POINT('Ctrl Pts',(-23.5790256782679,-84.784902956671,
81.090859097905));
#180321=CARTESIAN_POINT('Ctrl Pts',(-23.4896506782679,-86.79940000028,77.696372653464));
#180322=CARTESIAN_POINT('Ctrl Pts',(-23.4002756782679,-87.67474575053,73.8474109262253));
#180323=CARTESIAN_POINT('Ctrl Pts',(-23.3109006782679,-87.32643156769,69.915564821625));
#180324=CARTESIAN_POINT('Ctrl Pts',(-23.2215256782679,-85.78808480163,66.280427164319));
#180325=CARTESIAN_POINT('Ctrl Pts',(-23.1321506782679,-83.208222301335,
63.292945609594));
#180326=CARTESIAN_POINT('Ctrl Pts',(-23.0427756782679,-79.835912129926,
61.24154104977));
#180327=CARTESIAN_POINT('Ctrl Pts',(-22.9534006782679,-75.9967277481947,
60.32426255155));
#180328=CARTESIAN_POINT('Ctrl Pts',(-22.8640256782679,-72.061316125801,
60.62966707439));
#180329=CARTESIAN_POINT('Ctrl Pts',(-22.7746506782679,-68.409614313737,
62.12826990236));
#180330=CARTESIAN_POINT('Ctrl Pts',(-22.6852756782679,-65.394169123036,
64.675391191609));
#180331=CARTESIAN_POINT('Ctrl Pts',(-22.5959006782679,-63.30610114364,68.0251238188));
#180332=CARTESIAN_POINT('Ctrl Pts',(-22.5065256782679,-62.34699904441,71.854074030477));
#180333=CARTESIAN_POINT('Ctrl Pts',(-22.4171506782679,-62.60945756717,75.792582896034));
#180334=CARTESIAN_POINT('Ctrl Pts',(-22.3277756782679,-64.06813813831,79.460414346857));
#180335=CARTESIAN_POINT('Ctrl Pts',(-22.2384006782679,-66.582215134543,
82.503464365711));
#180336=CARTESIAN_POINT('Ctrl Pts',(-22.1490256782679,-69.908971632833,
84.62794730547));
#180337=CARTESIAN_POINT('Ctrl Pts',(-22.0596506782679,-73.727232067669,
85.62875888215));
#180338=CARTESIAN_POINT('Ctrl Pts',(-21.9702756782679,-77.668369533221,
85.4092775894));
#180339=CARTESIAN_POINT('Ctrl Pts',(-21.8809006782679,-81.351894187539,
83.99069284351));
#180340=CARTESIAN_POINT('Ctrl Pts',(-21.7915256782679,-84.422186942024,
81.509959290305));
#180341=CARTESIAN_POINT('Ctrl Pts',(-21.7021506782679,-86.58283204993,78.206574771673));
#180342=CARTESIAN_POINT('Ctrl Pts',(-21.6127756782679,-87.62523401748,74.399458448487));
#180343=CARTESIAN_POINT('Ctrl Pts',(-21.5234006782689,-87.44875607083,70.456161338886));
#180344=CARTESIAN_POINT('Ctrl Pts',(-21.4340256782689,-86.07043594758,66.757381783671));
#180345=CARTESIAN_POINT('Ctrl Pts',(-21.3446506782689,-83.623341019893,
63.660211627688));
#180346=CARTESIAN_POINT('Ctrl Pts',(-21.2552756782689,-80.343721550643,
61.4636614468));
#180347=CARTESIAN_POINT('Ctrl Pts',(-21.1659006782689,-76.548202347877,
60.37979312378));
#180348=CARTESIAN_POINT('Ctrl Pts',(-21.0765256782689,-72.603214807152,
60.51324672522));
#180349=CARTESIAN_POINT('Ctrl Pts',(-20.9871506782689,-68.889620468817,
61.85113821951));
#180350=CARTESIAN_POINT('Ctrl Pts',(-20.8977756782689,-65.765941443611,
64.264303341857));
#180351=CARTESIAN_POINT('Ctrl Pts',(-20.8084006782689,-63.53374755725,67.519767519802));
#180352=CARTESIAN_POINT('Ctrl Pts',(-20.7190256782689,-62.40854184824,71.303237973316));
#180353=CARTESIAN_POINT('Ctrl Pts',(-20.6296506782689,-62.49895522482,75.2494465311));
#180354=CARTESIAN_POINT('Ctrl Pts',(-20.5402756782689,-63.79625889445,78.977413771966));
#180355=CARTESIAN_POINT('Ctrl Pts',(-20.4509006782689,-66.175207068926,
82.127229979831));
#180356=CARTESIAN_POINT('Ctrl Pts',(-20.3615256782689,-69.406128587882,
84.39480196293));
#180357=CARTESIAN_POINT('Ctrl Pts',(-20.2721506782689,-73.177100096994,
85.5612111697));
#180358=CARTESIAN_POINT('Ctrl Pts',(-20.1827756782689,-77.124060112478,
85.51384877627));
#180359=CARTESIAN_POINT('Ctrl Pts',(-20.0934006782689,-80.865956665065,
84.25728729746));
#180360=CARTESIAN_POINT('Ctrl Pts',(-20.0040256782689,-84.041535258926,
81.912839141965));
#180361=CARTESIAN_POINT('Ctrl Pts',(-19.9146506782689,-86.34421552051,78.706844729098));
#180362=CARTESIAN_POINT('Ctrl Pts',(-19.8252756782689,-87.5516894335,74.948820873245));
#180363=CARTESIAN_POINT('Ctrl Pts',(-19.7359006782689,-87.54738366077,71.001579045262));
#180364=CARTESIAN_POINT('Ctrl Pts',(-19.6465256782689,-86.331713884,67.246198442551));
#180365=CARTESIAN_POINT('Ctrl Pts',(-19.5571506782689,-84.022044739653,
64.045235275048));
#180366=CARTESIAN_POINT('Ctrl Pts',(-19.4677756782689,-80.841358816111,
61.70772091653));
#180367=CARTESIAN_POINT('Ctrl Pts',(-19.3784006782689,-77.096730146679,
60.45932528185));
#180368=CARTESIAN_POINT('Ctrl Pts',(-19.2890256782679,-73.149674822947,
60.42057650697));
#180369=CARTESIAN_POINT('Ctrl Pts',(-19.1996506782679,-69.381262119169,
61.59520028015));
#180370=CARTESIAN_POINT('Ctrl Pts',(-19.1102756782679,-66.155276240892,
63.869851596353));
#180371=CARTESIAN_POINT('Ctrl Pts',(-19.0506923449349,-64.57394335288,65.973094643852));
#180372=CARTESIAN_POINT('Ctrl Pts',(-19.0209006782679,-63.9637045108,67.120786984341));
#180373=CARTESIAN_POINT('Ctrl Pts',(-24.8977186478319,-75.4467352742876,
60.19606492144));
#180374=CARTESIAN_POINT('Ctrl Pts',(-24.8679269811659,-74.1163770334926,
60.14960778797));
#180375=CARTESIAN_POINT('Ctrl Pts',(-24.8083436478319,-71.441294398629,
60.47512121458));
#180376=CARTESIAN_POINT('Ctrl Pts',(-24.7189686478319,-67.772045047785,
62.1715032276));
#180377=CARTESIAN_POINT('Ctrl Pts',(-24.6295936478319,-64.80065726501,64.912231636138));
#180378=CARTESIAN_POINT('Ctrl Pts',(-24.5402186478319,-62.81393226732,68.432705572515));
#180379=CARTESIAN_POINT('Ctrl Pts',(-24.4508436478319,-62.00369241884,72.393047995661));
#180380=CARTESIAN_POINT('Ctrl Pts',(-24.3614686478319,-62.44815609648,76.41091479114));
#180381=CARTESIAN_POINT('Ctrl Pts',(-24.2720936478319,-64.10441464328,80.098408469768));
#180382=CARTESIAN_POINT('Ctrl Pts',(-24.1827186478319,-66.812567295151,
83.09952674895));
#180383=CARTESIAN_POINT('Ctrl Pts',(-24.0933436478319,-70.311160544158,
85.12453220716));
#180384=CARTESIAN_POINT('Ctrl Pts',(-24.0039686478319,-74.2624291384833,
85.97792442938));
#180385=CARTESIAN_POINT('Ctrl Pts',(-23.9145936478319,-78.284905151586,
85.57731423897));
#180386=CARTESIAN_POINT('Ctrl Pts',(-23.8252186478319,-81.99024605983,83.96137780724));
#180387=CARTESIAN_POINT('Ctrl Pts',(-23.7358436478319,-85.02072656512,81.286122734268));
#180388=CARTESIAN_POINT('Ctrl Pts',(-23.6464686478319,-87.08377452069,77.809826583006));
#180389=CARTESIAN_POINT('Ctrl Pts',(-23.5570936478319,-87.98021676974,73.8681019487347));
#180390=CARTESIAN_POINT('Ctrl Pts',(-23.4677186478319,-87.62350794999,69.841495360525));
#180391=CARTESIAN_POINT('Ctrl Pts',(-23.3783436478319,-86.04808585604,66.118748119013));
#180392=CARTESIAN_POINT('Ctrl Pts',(-23.2889686478319,-83.406046705982,
63.059265985079));
#180393=CARTESIAN_POINT('Ctrl Pts',(-23.1995936478319,-79.952461292809,
60.95842101407));
#180394=CARTESIAN_POINT('Ctrl Pts',(-23.1102186478319,-76.020749645512,
60.01903540591));
#180395=CARTESIAN_POINT('Ctrl Pts',(-23.0208436478319,-71.990491607817,
60.33180041019));
#180396=CARTESIAN_POINT('Ctrl Pts',(-22.9314686478319,-68.250781002811,
61.8665207069));
#180397=CARTESIAN_POINT('Ctrl Pts',(-22.8420936478319,-65.162661287992,
64.475029557805));
#180398=CARTESIAN_POINT('Ctrl Pts',(-22.7527186478319,-63.02426928109,67.905493290763));
#180399=CARTESIAN_POINT('Ctrl Pts',(-22.6633436478319,-62.04205209131,71.826724116717));
#180400=CARTESIAN_POINT('Ctrl Pts',(-22.5739686478319,-62.31083606423,75.860154043494));
#180401=CARTESIAN_POINT('Ctrl Pts',(-22.4845936478319,-63.80467194732,79.616383023829));
#180402=CARTESIAN_POINT('Ctrl Pts',(-22.3952186478319,-66.379340112613,
82.732772864167));
#180403=CARTESIAN_POINT('Ctrl Pts',(-22.3058436478319,-69.786273974476,
84.90845745969));
#180404=CARTESIAN_POINT('Ctrl Pts',(-22.2164686478319,-73.696557391833,
85.93338935707));
#180405=CARTESIAN_POINT('Ctrl Pts',(-22.1270936478319,-77.732679269865,
85.70861839811));
#180406=CARTESIAN_POINT('Ctrl Pts',(-22.0377186478319,-81.504979671842,
84.25584468017));
#180407=CARTESIAN_POINT('Ctrl Pts',(-21.9483436478319,-84.649268818474,
81.715323560263));
#180408=CARTESIAN_POINT('Ctrl Pts',(-21.8589686478319,-86.86198711791,78.332324960555));
#180409=CARTESIAN_POINT('Ctrl Pts',(-21.7695936478319,-87.92951176624,74.43345423642));
#180410=CARTESIAN_POINT('Ctrl Pts',(-21.6802186478319,-87.74878056675,70.395120665275));
#180411=CARTESIAN_POINT('Ctrl Pts',(-21.5908436478319,-86.3372418795,66.607197707679));
#180412=CARTESIAN_POINT('Ctrl Pts',(-21.5014686478319,-83.831170101586,
63.435383393718));
#180413=CARTESIAN_POINT('Ctrl Pts',(-21.4120936478329,-80.472509307037,
61.18589468171));
#180414=CARTESIAN_POINT('Ctrl Pts',(-21.3227186478329,-76.585515202752,
60.07590430719));
#180415=CARTESIAN_POINT('Ctrl Pts',(-21.2333436478329,-72.545450459805,
60.212574242));
#180416=CARTESIAN_POINT('Ctrl Pts',(-21.1439686478329,-68.742355671542,
61.58270993957));
#180417=CARTESIAN_POINT('Ctrl Pts',(-21.0545936478329,-65.543393604434,
64.054034178009));
#180418=CARTESIAN_POINT('Ctrl Pts',(-20.9652186478329,-63.25740214652,67.387957520349));
#180419=CARTESIAN_POINT('Ctrl Pts',(-20.8758436478329,-62.10507812355,71.262612491355));
#180420=CARTESIAN_POINT('Ctrl Pts',(-20.7864686478329,-62.19767053133,75.3039276788));
#180421=CARTESIAN_POINT('Ctrl Pts',(-20.6970936478329,-63.52624020677,79.121741767484));
#180422=CARTESIAN_POINT('Ctrl Pts',(-20.6077186478329,-65.96252284285,82.347470943245));
#180423=CARTESIAN_POINT('Ctrl Pts',(-20.5183436478329,-69.271312029438,
84.66969313695));
#180424=CARTESIAN_POINT('Ctrl Pts',(-20.4289686478329,-73.133166821969,
85.86421369334));
#180425=CARTESIAN_POINT('Ctrl Pts',(-20.3395936478329,-77.175251577815,
85.81570983017));
#180426=CARTESIAN_POINT('Ctrl Pts',(-20.2502186478329,-81.007330685234,
84.52886426336));
#180427=CARTESIAN_POINT('Ctrl Pts',(-20.1608436478329,-84.259443140101,
82.127913122978));
#180428=CARTESIAN_POINT('Ctrl Pts',(-20.0714686478329,-86.61761974852,78.844651804709));
#180429=CARTESIAN_POINT('Ctrl Pts',(-19.9820936478329,-87.85419470181,74.996056713737));
#180430=CARTESIAN_POINT('Ctrl Pts',(-19.8927186478329,-87.84978515668,70.953683353497));
#180431=CARTESIAN_POINT('Ctrl Pts',(-19.8033436478329,-86.60481681305,67.107795220083));
#180432=CARTESIAN_POINT('Ctrl Pts',(-19.7139686478329,-84.239482884453,
63.829686404028));
#180433=CARTESIAN_POINT('Ctrl Pts',(-19.6245936478329,-80.982140009367,
61.43583617042));
#180434=CARTESIAN_POINT('Ctrl Pts',(-19.5352186478319,-77.147262939005,
60.15735325081));
#180435=CARTESIAN_POINT('Ctrl Pts',(-19.4458436478319,-73.105080577911,
60.11767060096));
#180436=CARTESIAN_POINT('Ctrl Pts',(-19.3564686478319,-69.245846259876,
61.32060370107));
#180437=CARTESIAN_POINT('Ctrl Pts',(-19.2670936478319,-65.94211166667,63.650075845204));
#180438=CARTESIAN_POINT('Ctrl Pts',(-19.2075103144989,-64.32266745252,65.804008650901));
#180439=CARTESIAN_POINT('Ctrl Pts',(-19.1777186478319,-63.6977213899,66.979361250291));
#180440=CARTESIAN_POINT('Ctrl Pts',(-25.0545366173959,-75.4572485563053,
59.89500391474));
#180441=CARTESIAN_POINT('Ctrl Pts',(-25.0247449507299,-74.0955822183551,
59.84745347843));
#180442=CARTESIAN_POINT('Ctrl Pts',(-24.9651616173959,-71.357545302109,
60.18062740255));
#180443=CARTESIAN_POINT('Ctrl Pts',(-24.8757866173959,-67.601945364152,
61.91693136384));
#180444=CARTESIAN_POINT('Ctrl Pts',(-24.7864116173959,-64.56063017797,64.722158934074));
#180445=CARTESIAN_POINT('Ctrl Pts',(-24.6970366173959,-62.52715042104,68.325482238879));
#180446=CARTESIAN_POINT('Ctrl Pts',(-24.6076616173959,-61.69784272518,72.379025712351));
#180447=CARTESIAN_POINT('Ctrl Pts',(-24.5182866173959,-62.15276622603,76.491447312794));
#180448=CARTESIAN_POINT('Ctrl Pts',(-24.4289116173959,-63.84800247215,80.265720932952));
#180449=CARTESIAN_POINT('Ctrl Pts',(-24.3395366173959,-66.619887661413,
83.33746628068));
#180450=CARTESIAN_POINT('Ctrl Pts',(-24.2501616173959,-70.200815347859,
85.41012737455));
#180451=CARTESIAN_POINT('Ctrl Pts',(-24.1607866173959,-74.2450714527985,
86.28360297416));
#180452=CARTESIAN_POINT('Ctrl Pts',(-24.0714116173959,-78.362210742274,
85.87356499026));
#180453=CARTESIAN_POINT('Ctrl Pts',(-23.9820366173959,-82.154751601322,
84.21959978308));
#180454=CARTESIAN_POINT('Ctrl Pts',(-23.8926616173959,-85.25655017356,81.481386370637));
#180455=CARTESIAN_POINT('Ctrl Pts',(-23.8032866173959,-87.3681490411,77.923280512555));
#180456=CARTESIAN_POINT('Ctrl Pts',(-23.7139116173959,-88.28568778894,73.8887929712528));
#180457=CARTESIAN_POINT('Ctrl Pts',(-23.6245366173959,-87.92058433229,69.767425899435));
#180458=CARTESIAN_POINT('Ctrl Pts',(-23.5351616173959,-86.30808691046,65.957069073716));
#180459=CARTESIAN_POINT('Ctrl Pts',(-23.4457866173959,-83.603871110638,
62.82558636057));
#180460=CARTESIAN_POINT('Ctrl Pts',(-23.3564116173959,-80.069010455704,
60.67530097837));
#180461=CARTESIAN_POINT('Ctrl Pts',(-23.2670366173959,-76.044771542844,
59.71380826027));
#180462=CARTESIAN_POINT('Ctrl Pts',(-23.1776616173959,-71.919667089848,
60.03393374599));
#180463=CARTESIAN_POINT('Ctrl Pts',(-23.0882866173959,-68.091947691899,
61.60477151142));
#180464=CARTESIAN_POINT('Ctrl Pts',(-22.9989116173959,-64.93115345296,64.274667923988));
#180465=CARTESIAN_POINT('Ctrl Pts',(-22.9095366173959,-62.74243741855,67.785862762707));
#180466=CARTESIAN_POINT('Ctrl Pts',(-22.8201616173959,-61.73710513821,71.799374202937));
#180467=CARTESIAN_POINT('Ctrl Pts',(-22.7307866173959,-62.01221456129,75.927725190932));
#180468=CARTESIAN_POINT('Ctrl Pts',(-22.6414116173959,-63.54120575633,79.77235170078));
#180469=CARTESIAN_POINT('Ctrl Pts',(-22.5520366173959,-66.176465090666,
82.962081362607));
#180470=CARTESIAN_POINT('Ctrl Pts',(-22.4626616173959,-69.663576316097,
85.1889676139));
#180471=CARTESIAN_POINT('Ctrl Pts',(-22.3732866173959,-73.665882715971,
86.23801983199));
#180472=CARTESIAN_POINT('Ctrl Pts',(-22.2839116173959,-77.796989006481,
86.00795920683));
#180473=CARTESIAN_POINT('Ctrl Pts',(-22.1945366173959,-81.65806515612,84.52099651684));
#180474=CARTESIAN_POINT('Ctrl Pts',(-22.1051616173959,-84.876350694903,
81.920687830243));
#180475=CARTESIAN_POINT('Ctrl Pts',(-22.0157866173959,-87.14114218589,78.458075149464));
#180476=CARTESIAN_POINT('Ctrl Pts',(-21.9264116173959,-88.233789515,74.467450024384));
#180477=CARTESIAN_POINT('Ctrl Pts',(-21.8370366173959,-88.04880506268,70.334079991696));
#180478=CARTESIAN_POINT('Ctrl Pts',(-21.7476616173959,-86.60404781143,66.457013631716));
#180479=CARTESIAN_POINT('Ctrl Pts',(-21.6582866173959,-84.038999183303,
63.210555159771));
#180480=CARTESIAN_POINT('Ctrl Pts',(-21.5689116173959,-80.601297063461,
60.90812791663));
#180481=CARTESIAN_POINT('Ctrl Pts',(-21.4795366173959,-76.622828057659,
59.7720154906));
#180482=CARTESIAN_POINT('Ctrl Pts',(-21.3901616173959,-72.487686112493,
59.91190175878));
#180483=CARTESIAN_POINT('Ctrl Pts',(-21.3007866173969,-68.595090874297,
61.31428165962));
#180484=CARTESIAN_POINT('Ctrl Pts',(-21.2114116173969,-65.320845765281,
63.843765014137));
#180485=CARTESIAN_POINT('Ctrl Pts',(-21.1220366173969,-62.9810567358,67.256147520865));
#180486=CARTESIAN_POINT('Ctrl Pts',(-21.0326616173969,-61.80161439886,71.22198700936));
#180487=CARTESIAN_POINT('Ctrl Pts',(-20.9432866173969,-61.89638583783,75.358408826466));
#180488=CARTESIAN_POINT('Ctrl Pts',(-20.8539116173969,-63.25622151907,79.266069762973));
#180489=CARTESIAN_POINT('Ctrl Pts',(-20.7645366173969,-65.74983861675,82.567711906636));
#180490=CARTESIAN_POINT('Ctrl Pts',(-20.6751616173969,-69.136495470965,
84.94458431096));
#180491=CARTESIAN_POINT('Ctrl Pts',(-20.5857866173969,-73.089233546913,
86.16721621697));
#180492=CARTESIAN_POINT('Ctrl Pts',(-20.4964116173969,-77.226443043123,
86.11757088408));
#180493=CARTESIAN_POINT('Ctrl Pts',(-20.4070366173969,-81.148704705378,
84.80044122928));
#180494=CARTESIAN_POINT('Ctrl Pts',(-20.3176616173969,-84.477351021258,
82.34298710401));
#180495=CARTESIAN_POINT('Ctrl Pts',(-20.2282866173969,-86.89102397653,78.982458880342));
#180496=CARTESIAN_POINT('Ctrl Pts',(-20.1389116173969,-88.15669997012,75.043292554251));
#180497=CARTESIAN_POINT('Ctrl Pts',(-20.0495366173969,-88.15218665258,70.905787661752));
#180498=CARTESIAN_POINT('Ctrl Pts',(-19.9601616173959,-86.87791974211,66.969391997631));
#180499=CARTESIAN_POINT('Ctrl Pts',(-19.8707866173959,-84.456921029265,
63.614137533019));
#180500=CARTESIAN_POINT('Ctrl Pts',(-19.7814116173959,-81.122921202634,
61.16395142431));
#180501=CARTESIAN_POINT('Ctrl Pts',(-19.6920366173959,-77.19779573134,59.85538121976));
#180502=CARTESIAN_POINT('Ctrl Pts',(-19.6026616173959,-73.060486332881,
59.81476469495));
#180503=CARTESIAN_POINT('Ctrl Pts',(-19.5132866173959,-69.110430400585,
61.04600712199));
#180504=CARTESIAN_POINT('Ctrl Pts',(-19.4239116173959,-65.728947092448,
63.430300094054));
#180505=CARTESIAN_POINT('Ctrl Pts',(-19.3643282840629,-64.07139155217,65.634922657953));
#180506=CARTESIAN_POINT('Ctrl Pts',(-19.3345366173959,-63.431738269,66.837935516246));
#180507=CARTESIAN_POINT('Ctrl Pts',(-19.0011309998534,-67.124599619487,
63.6058883503008));
#180508=CARTESIAN_POINT('Ctrl Pts',(-19.0704950559586,-67.0389239813991,
63.5038382415724));
#180509=CARTESIAN_POINT('Ctrl Pts',(-19.1398591185752,-66.95324791439,63.4017884768216));
#180510=CARTESIAN_POINT('Ctrl Pts',(-19.2784798392654,-66.7820276024722,
63.197847668815));
#180511=CARTESIAN_POINT('Ctrl Pts',(-19.3477365383098,-66.6964833082578,
63.0959565641899));
#180512=CARTESIAN_POINT('Ctrl Pts',(-19.4169932345698,-66.6109385987686,
62.9940658153934));
#180513=CARTESIAN_POINT('',(-24.5011471556111,-70.8102632894868,61.4776867539786));
#180514=CARTESIAN_POINT('Ctrl Pts',(-18.9799062324529,-67.340715181151,
63.474668109995));
#180515=CARTESIAN_POINT('Ctrl Pts',(-18.9294356932999,-65.751498900725,
64.932060456454));
#180516=CARTESIAN_POINT('Ctrl Pts',(-18.8284946149979,-63.4247304556,68.654743887637));
#180517=CARTESIAN_POINT('Ctrl Pts',(-18.7275535366989,-63.30638992216,72.8921974616309));
#180518=CARTESIAN_POINT('Ctrl Pts',(-18.6770829975479,-63.77070234627,74.847875926051));
#180519=CARTESIAN_POINT('Ctrl Pts',(-19.1367242020169,-67.151809631229,
63.240013146138));
#180520=CARTESIAN_POINT('Ctrl Pts',(-19.0862536628639,-65.521252914769,
64.730686006568));
#180521=CARTESIAN_POINT('Ctrl Pts',(-18.9853125845619,-63.12987316536,68.542252716656));
#180522=CARTESIAN_POINT('Ctrl Pts',(-18.8843715062629,-63.00052245572,72.8890389661518));
#180523=CARTESIAN_POINT('Ctrl Pts',(-18.8339009671119,-63.47350284263,74.897076676965));
#180524=CARTESIAN_POINT('Ctrl Pts',(-19.2935421715809,-66.962904081306,
63.005358182281));
#180525=CARTESIAN_POINT('Ctrl Pts',(-19.2430716324269,-65.291006928818,
64.529311556686));
#180526=CARTESIAN_POINT('Ctrl Pts',(-19.1421305541259,-62.83501587512,68.429761545683));
#180527=CARTESIAN_POINT('Ctrl Pts',(-19.0411894758269,-62.6946549893,72.8858804706761));
#180528=CARTESIAN_POINT('Ctrl Pts',(-18.9907189366759,-63.176303339,74.94627742788));
#180529=CARTESIAN_POINT('Ctrl Pts',(-19.4503601411449,-66.773998531384,
62.77070321842));
#180530=CARTESIAN_POINT('Ctrl Pts',(-19.3998896019909,-65.060760942862,
64.327937106799));
#180531=CARTESIAN_POINT('Ctrl Pts',(-19.2989485236899,-62.54015858487,68.317270374702));
#180532=CARTESIAN_POINT('Ctrl Pts',(-19.1980074453909,-62.38878752287,72.8827219751971));
#180533=CARTESIAN_POINT('Ctrl Pts',(-19.1475369062399,-62.87910383536,74.995478178794));
#180534=CARTESIAN_POINT('Ctrl Pts',(-19.4175174361239,-66.6110703651319,
62.9926155500965));
#180535=CARTESIAN_POINT('Ctrl Pts',(-19.4032204672389,-66.137812315149,
63.4414112721957));
#180536=CARTESIAN_POINT('Ctrl Pts',(-19.3888608262407,-65.6990094831001,
63.9263196278806));
#180537=CARTESIAN_POINT('Ctrl Pts',(-19.3744395805111,-65.2989377577199,
64.4413732029171));
#180538=CARTESIAN_POINT('Ctrl Pts',(-19.3705423958786,-65.190822730123,
64.580560823402));
#180539=CARTESIAN_POINT('Ctrl Pts',(-19.3666407123033,-65.0855363738124,
64.7219496850546));
#180540=CARTESIAN_POINT('Ctrl Pts',(-19.3627345508503,-64.9831634543278,
64.8654214859086));
#180541=CARTESIAN_POINT('Ctrl Pts',(-19.3583084311856,-64.8671634380688,
65.0279911509681));
#180542=CARTESIAN_POINT('Ctrl Pts',(-19.3538768656123,-64.7549293313154,
65.1931996793288));
#180543=CARTESIAN_POINT('Ctrl Pts',(-19.3494392777582,-64.6465764817334,
65.3608767801899));
#180544=CARTESIAN_POINT('Ctrl Pts',(-19.3423986111131,-64.4746641007192,
65.6269128813334));
#180545=CARTESIAN_POINT('Ctrl Pts',(-19.3353359681682,-64.3125383180186,
65.8991738812957));
#180546=CARTESIAN_POINT('Ctrl Pts',(-19.3282589746446,-64.1606418137509,
66.1769664936579));
#180547=CARTESIAN_POINT('Ctrl Pts',(-19.321308349306,-64.0114576032676,
66.4497987866271));
#180548=CARTESIAN_POINT('Ctrl Pts',(-19.3143438813066,-63.8721403447319,
66.7279675738643));
#180549=CARTESIAN_POINT('Ctrl Pts',(-19.3073727951192,-63.7431498331095,
67.0108436589339));
#180550=CARTESIAN_POINT('Ctrl Pts',(-19.2983245975766,-63.5757251880965,
67.3780057666716));
#180551=CARTESIAN_POINT('Ctrl Pts',(-19.289246402415,-63.4254515690211,
67.7536630696148));
#180552=CARTESIAN_POINT('Ctrl Pts',(-19.2801213645055,-63.2937354273005,
68.136063387383));
#180553=CARTESIAN_POINT('Ctrl Pts',(-19.2782027682036,-63.2660412845564,
68.2164654462903));
#180554=CARTESIAN_POINT('Ctrl Pts',(-19.2762821010918,-63.2391674508634,
68.297165429793));
#180555=CARTESIAN_POINT('Ctrl Pts',(-19.2743592065957,-63.2131268729228,
68.3781467925786));
#180556=CARTESIAN_POINT('Ctrl Pts',(-19.2735558745621,-63.2022478410906,
68.4119785618106));
#180557=CARTESIAN_POINT('Ctrl Pts',(-19.272751612069,-63.1915151897248,
68.445859771803));
#180558=CARTESIAN_POINT('Ctrl Pts',(-19.2719468277686,-63.180929072759,
68.4797889760641));
#180559=CARTESIAN_POINT('Ctrl Pts',(-19.2713566720993,-63.1731661766147,
68.5046695710727));
#180560=CARTESIAN_POINT('Ctrl Pts',(-19.270766235899,-63.1654820780196,
68.5295759752021));
#180561=CARTESIAN_POINT('Ctrl Pts',(-19.2701755446975,-63.1578768357417,
68.5545076247395));
#180562=CARTESIAN_POINT('Ctrl Pts',(-19.2583305133496,-63.0053701910583,
69.0544578010007));
#180563=CARTESIAN_POINT('Ctrl Pts',(-19.2464062952225,-62.8846459609022,
69.5643192941634));
#180564=CARTESIAN_POINT('Ctrl Pts',(-19.2344955395952,-62.7961070134394,
70.0794616457634));
#180565=CARTESIAN_POINT('Ctrl Pts',(-19.2255648541586,-62.7297205041846,
70.4657154185047));
#180566=CARTESIAN_POINT('Ctrl Pts',(-19.2166306713089,-62.6813849908161,
70.8551919742191));
#180567=CARTESIAN_POINT('Ctrl Pts',(-19.2076647208652,-62.6513402357164,
71.2459541183865));
#180568=CARTESIAN_POINT('Ctrl Pts',(-19.2044523919758,-62.6405757735006,
71.3859567352259));
#180569=CARTESIAN_POINT('Ctrl Pts',(-19.2012374970565,-62.6321654850941,
71.5260384699883));
#180570=CARTESIAN_POINT('Ctrl Pts',(-19.1980166927661,-62.6261114628072,
71.666139079149));
#180571=CARTESIAN_POINT('Ctrl Pts',(-19.1933795896618,-62.6173952779637,
71.8678467617854));
#180572=CARTESIAN_POINT('Ctrl Pts',(-19.1887351237908,-62.6135660108167,
72.0695940567608));
#180573=CARTESIAN_POINT('Ctrl Pts',(-19.1840873605703,-62.6145893742609,
72.2711996352988));
#180574=CARTESIAN_POINT('Ctrl Pts',(-19.1794322607379,-62.6156143531102,
72.4731234533451));
#180575=CARTESIAN_POINT('Ctrl Pts',(-19.174773853138,-62.6215072801478,
72.6749059000198));
#180576=CARTESIAN_POINT('Ctrl Pts',(-19.1701162224702,-62.6322855183008,
72.8763672965785));
#180577=CARTESIAN_POINT('Ctrl Pts',(-19.1691220913338,-62.6345860403706,
72.9193674959065));
#180578=CARTESIAN_POINT('Ctrl Pts',(-19.1681279955922,-62.6371093117162,
72.9623530532898));
#180579=CARTESIAN_POINT('Ctrl Pts',(-19.1671339749643,-62.6398558076609,
73.00532218268));
#180580=CARTESIAN_POINT('Ctrl Pts',(-19.164564094539,-62.6469564310972,
73.1164119542729));
#180581=CARTESIAN_POINT('Ctrl Pts',(-19.1619911494633,-62.6555521718381,
73.227443772742));
#180582=CARTESIAN_POINT('Ctrl Pts',(-19.1594114054907,-62.6656570955864,
73.3383711450185));
#180583=CARTESIAN_POINT('Ctrl Pts',(-19.1547191646527,-62.6840367240996,
73.5401345571109));
#180584=CARTESIAN_POINT('Ctrl Pts',(-19.1500219576314,-62.7073564942426,
73.741558755367));
#180585=CARTESIAN_POINT('Ctrl Pts',(-19.1453140801805,-62.7357018617097,
73.9423640348264));
#180586=CARTESIAN_POINT('Ctrl Pts',(-19.1406652548524,-62.7636916859117,
74.1406505618012));
#180587=CARTESIAN_POINT('Ctrl Pts',(-19.1360060250999,-62.7965818773787,
74.3383335923708));
#180588=CARTESIAN_POINT('Ctrl Pts',(-19.1313308986451,-62.8344042122621,
74.5351501297222));
#180589=CARTESIAN_POINT('Ctrl Pts',(-19.1296852922034,-62.8477173661469,
74.6044279481571));
#180590=CARTESIAN_POINT('Ctrl Pts',(-19.1280377161879,-62.8616411390047,
74.6735984677276));
#180591=CARTESIAN_POINT('Ctrl Pts',(-19.1263879310737,-62.8761753834789,
74.7426504105179));
#180592=CARTESIAN_POINT('Ctrl Pts',(-19.7210834129279,-66.6679911229052,
62.9389668654546));
#180593=CARTESIAN_POINT('Ctrl Pts',(-19.0031848503602,-66.6679911229052,
62.9389668654546));
#180594=CARTESIAN_POINT('Ctrl Pts',(-19.7210834129279,-65.8978577481411,
63.6603901351978));
#180595=CARTESIAN_POINT('Ctrl Pts',(-19.0031848503602,-65.8978577481411,
63.6603901351978));
#180596=CARTESIAN_POINT('Ctrl Pts',(-19.7210834129279,-65.2182108438486,
64.4762669802466));
#180597=CARTESIAN_POINT('Ctrl Pts',(-19.0031848503602,-65.2182108438486,
64.4762669802466));
#180598=CARTESIAN_POINT('Ctrl Pts',(-19.7210834129279,-64.0409039909203,
66.2981609192099));
#180599=CARTESIAN_POINT('Ctrl Pts',(-19.0031848503602,-64.0409039909203,
66.2981609192099));
#180600=CARTESIAN_POINT('Ctrl Pts',(-19.7210834129279,-63.5546993668503,
67.315919751713));
#180601=CARTESIAN_POINT('Ctrl Pts',(-19.0031848503602,-63.5546993668503,
67.315919751713));
#180602=CARTESIAN_POINT('Ctrl Pts',(-19.7210834129279,-62.8715543789953,
69.4403738334441));
#180603=CARTESIAN_POINT('Ctrl Pts',(-19.0031848503602,-62.8715543789953,
69.4403738334441));
#180604=CARTESIAN_POINT('Ctrl Pts',(-19.7210834129279,-62.6742843975167,
70.5513335535036));
#180605=CARTESIAN_POINT('Ctrl Pts',(-19.0031848503602,-62.6742843975167,
70.5513335535036));
#180606=CARTESIAN_POINT('Ctrl Pts',(-19.7210834129279,-62.6020249954524,
72.2235418419717));
#180607=CARTESIAN_POINT('Ctrl Pts',(-19.0031848503602,-62.6020249954524,
72.2235418419717));
#180608=CARTESIAN_POINT('Ctrl Pts',(-19.7210834129279,-62.6151667392939,
72.7841104016103));
#180609=CARTESIAN_POINT('Ctrl Pts',(-19.0031848503602,-62.6151667392939,
72.7841104016103));
#180610=CARTESIAN_POINT('Ctrl Pts',(-19.7210834129279,-62.7109382443801,
73.8354475183249));
#180611=CARTESIAN_POINT('Ctrl Pts',(-19.0031848503602,-62.7109382443801,
73.8354475183249));
#180612=CARTESIAN_POINT('Ctrl Pts',(-19.7210834129279,-62.7860260362546,
74.3287972481997));
#180613=CARTESIAN_POINT('Ctrl Pts',(-19.0031848503602,-62.7860260362546,
74.3287972481997));
#180614=CARTESIAN_POINT('Ctrl Pts',(-19.7210834129279,-62.8923404913652,
74.8182427933889));
#180615=CARTESIAN_POINT('Ctrl Pts',(-19.0031848503602,-62.8923404913652,
74.8182427933889));
#180616=CARTESIAN_POINT('Ctrl Pts',(-19.7175219896827,-66.6111698442287,
62.9925212140073));
#180617=CARTESIAN_POINT('Ctrl Pts',(-19.7032357686158,-66.1380399280067,
63.4411857890246));
#180618=CARTESIAN_POINT('Ctrl Pts',(-19.6888822186527,-65.6993452916874,
63.9259433661227));
#180619=CARTESIAN_POINT('Ctrl Pts',(-19.6744617213196,-65.2993581486053,
64.4408320198377));
#180620=CARTESIAN_POINT('Ctrl Pts',(-19.6707792859395,-65.1972169551887,
64.5723145999073));
#180621=CARTESIAN_POINT('Ctrl Pts',(-19.6670924849657,-65.0976000062359,
64.7057617926725));
#180622=CARTESIAN_POINT('Ctrl Pts',(-19.6634013247513,-65.0005787608751,
64.8410738773966));
#180623=CARTESIAN_POINT('Ctrl Pts',(-19.6587526282975,-64.8783889091588,
65.0114877234196));
#180624=CARTESIAN_POINT('Ctrl Pts',(-19.6540986130407,-64.7603437515763,
65.1848208107002));
#180625=CARTESIAN_POINT('Ctrl Pts',(-19.6494392777599,-64.6465764817334,
65.3608767801898));
#180626=CARTESIAN_POINT('Ctrl Pts',(-19.6424230631589,-64.47526114775,65.6259889451786));
#180627=CARTESIAN_POINT('Ctrl Pts',(-19.6354021244996,-64.3136622764933,
65.8972863128408));
#180628=CARTESIAN_POINT('Ctrl Pts',(-19.6283648699486,-64.1622176497922,
66.1740854297641));
#180629=CARTESIAN_POINT('Ctrl Pts',(-19.6218433853392,-64.0218726054223,
66.4305975635544));
#180630=CARTESIAN_POINT('Ctrl Pts',(-19.6153078888229,-63.890248024282,
66.6918353088826));
#180631=CARTESIAN_POINT('Ctrl Pts',(-19.6087491550728,-63.7677253476843,
66.9572772307433));
#180632=CARTESIAN_POINT('Ctrl Pts',(-19.5999665130658,-63.603658189708,
67.3127240993296));
#180633=CARTESIAN_POINT('Ctrl Pts',(-19.5911412884054,-63.4558274535676,
67.675916413523));
#180634=CARTESIAN_POINT('Ctrl Pts',(-19.5822984309671,-63.3254298288066,
68.0451907172391));
#180635=CARTESIAN_POINT('Ctrl Pts',(-19.579653377898,-63.2864256223057,
68.1556471095548));
#180636=CARTESIAN_POINT('Ctrl Pts',(-19.5770067472021,-63.248980887577,
68.2666474635449));
#180637=CARTESIAN_POINT('Ctrl Pts',(-19.5743592065984,-63.2131268729228,
68.3781467925786));
#180638=CARTESIAN_POINT('Ctrl Pts',(-19.5735592697391,-63.2022938198484,
68.4118355764103));
#180639=CARTESIAN_POINT('Ctrl Pts',(-19.5727597867005,-63.1916069219557,
68.4455702452619));
#180640=CARTESIAN_POINT('Ctrl Pts',(-19.571960356956,-63.1810662645877,
68.4793492961659));
#180641=CARTESIAN_POINT('Ctrl Pts',(-19.5719568884247,-63.1810205312371,
68.4794958552583));
#180642=CARTESIAN_POINT('Ctrl Pts',(-19.5719534198934,-63.1809748006275,
68.4796424152244));
#180643=CARTESIAN_POINT('Ctrl Pts',(-19.5719499513622,-63.180929072759,
68.4797889760641));
#180644=CARTESIAN_POINT('Ctrl Pts',(-19.5599906187491,-63.0232615305662,
68.9851238653065));
#180645=CARTESIAN_POINT('Ctrl Pts',(-19.5480134164975,-62.8981803811709,
69.5008432106857));
#180646=CARTESIAN_POINT('Ctrl Pts',(-19.5359444704607,-62.806096716665,
70.0221345398778));
#180647=CARTESIAN_POINT('Ctrl Pts',(-19.5269013179855,-62.7370992568977,
70.4127334338935));
#180648=CARTESIAN_POINT('Ctrl Pts',(-19.5178062838736,-62.6865819724355,
70.8067205289833));
#180649=CARTESIAN_POINT('Ctrl Pts',(-19.5086971906096,-62.6547902527515,
71.2020880584462));
#180650=CARTESIAN_POINT('Ctrl Pts',(-19.5051350676615,-62.6423580587926,
71.3566970528696));
#180651=CARTESIAN_POINT('Ctrl Pts',(-19.5015738726351,-62.6327977573663,
71.511406589515));
#180652=CARTESIAN_POINT('Ctrl Pts',(-19.4980166927664,-62.6261114628072,
71.666139079149));
#180653=CARTESIAN_POINT('Ctrl Pts',(-19.4934105162437,-62.6174534094732,
71.8665014975118));
#180654=CARTESIAN_POINT('Ctrl Pts',(-19.4888065269332,-62.6136172626764,
72.066902646066));
#180655=CARTESIAN_POINT('Ctrl Pts',(-19.4841972065762,-62.6145695759266,
72.2671719933078));
#180656=CARTESIAN_POINT('Ctrl Pts',(-19.47958119344,-62.6155232719451,72.4677321336441));
#180657=CARTESIAN_POINT('Ctrl Pts',(-19.4749598337646,-62.6212793300511,
72.6681608772637));
#180658=CARTESIAN_POINT('Ctrl Pts',(-19.4703255764941,-62.6318559717216,
72.8682892798221));
#180659=CARTESIAN_POINT('Ctrl Pts',(-19.4694361642215,-62.6338858536111,
72.9066981654189));
#180660=CARTESIAN_POINT('Ctrl Pts',(-19.4685462768821,-62.6360934491295,
72.9450959748758));
#180661=CARTESIAN_POINT('Ctrl Pts',(-19.4676558610962,-62.6384791059619,
72.9834814859481));
#180662=CARTESIAN_POINT('Ctrl Pts',(-19.4649097591887,-62.64583663138,73.1018649724439));
#180663=CARTESIAN_POINT('Ctrl Pts',(-19.4621600849288,-62.6548904472578,
73.2201796537156));
#180664=CARTESIAN_POINT('Ctrl Pts',(-19.4594114054906,-62.6656570955864,
73.3383711450185));
#180665=CARTESIAN_POINT('Ctrl Pts',(-19.45468344815,-62.6841766265629,73.5416703443179));
#180666=CARTESIAN_POINT('Ctrl Pts',(-19.4499407562387,-62.7077104077423,
73.7446106609183));
#180667=CARTESIAN_POINT('Ctrl Pts',(-19.4451892350923,-62.7363450659676,
73.9469144504096));
#180668=CARTESIAN_POINT('Ctrl Pts',(-19.4404973026351,-62.7646206177726,
74.1466811539297));
#180669=CARTESIAN_POINT('Ctrl Pts',(-19.4357967610085,-62.7978699633399,
74.3458271887682));
#180670=CARTESIAN_POINT('Ctrl Pts',(-19.4310932961469,-62.8361259933756,
74.5440915419424));
#180671=CARTESIAN_POINT('Ctrl Pts',(-19.4295207442363,-62.848916477603,
74.6103790547806));
#180672=CARTESIAN_POINT('Ctrl Pts',(-19.4279478655588,-62.8622661963166,
74.676568064179));
#180673=CARTESIAN_POINT('Ctrl Pts',(-19.4263748726167,-62.8761750818273,
74.7426489773759));
#180674=CARTESIAN_POINT('Ctrl Pts',(-19.6963598728939,-66.773998531384,
62.77070321842));
#180675=CARTESIAN_POINT('Ctrl Pts',(-19.6458893337409,-65.060760942862,
64.327937106799));
#180676=CARTESIAN_POINT('Ctrl Pts',(-19.5449482554399,-62.54015858487,68.317270374702));
#180677=CARTESIAN_POINT('Ctrl Pts',(-19.4440071771409,-62.38878752287,72.8827219751971));
#180678=CARTESIAN_POINT('Ctrl Pts',(-19.3935366379889,-62.87910383536,74.995478178794));
#180679=CARTESIAN_POINT('Ctrl Pts',(-19.8531778424579,-66.962904081306,
63.005358182281));
#180680=CARTESIAN_POINT('Ctrl Pts',(-19.8027073033049,-65.291006928818,
64.529311556686));
#180681=CARTESIAN_POINT('Ctrl Pts',(-19.7017662250039,-62.83501587512,68.429761545683));
#180682=CARTESIAN_POINT('Ctrl Pts',(-19.6008251467039,-62.6946549893,72.8858804706761));
#180683=CARTESIAN_POINT('Ctrl Pts',(-19.5503546075529,-63.176303339,74.94627742788));
#180684=CARTESIAN_POINT('Ctrl Pts',(-20.0099958120219,-67.151809631229,
63.240013146138));
#180685=CARTESIAN_POINT('Ctrl Pts',(-19.9595252728689,-65.521252914769,
64.730686006568));
#180686=CARTESIAN_POINT('Ctrl Pts',(-19.8585841945679,-63.12987316536,68.542252716656));
#180687=CARTESIAN_POINT('Ctrl Pts',(-19.7576431162679,-63.00052245572,72.8890389661519));
#180688=CARTESIAN_POINT('Ctrl Pts',(-19.7071725771169,-63.47350284263,74.897076676965));
#180689=CARTESIAN_POINT('Ctrl Pts',(-20.1668137815859,-67.340715181151,
63.474668109995));
#180690=CARTESIAN_POINT('Ctrl Pts',(-20.1163432424329,-65.751498900725,
64.932060456454));
#180691=CARTESIAN_POINT('Ctrl Pts',(-20.0154021641319,-63.4247304556,68.654743887637));
#180692=CARTESIAN_POINT('Ctrl Pts',(-19.9144610858319,-63.30638992216,72.8921974616309));
#180693=CARTESIAN_POINT('Ctrl Pts',(-19.8639905466809,-63.77070234627,74.847875926051));
#180694=CARTESIAN_POINT('Ctrl Pts',(-19.7180890220136,-66.6111095357772,
62.994139891927));
#180695=CARTESIAN_POINT('Ctrl Pts',(-19.7872818346883,-66.6965738631944,
63.0959358861211));
#180696=CARTESIAN_POINT('Ctrl Pts',(-19.8564746631046,-66.7820377913851,
63.1977322539828));
#180697=CARTESIAN_POINT('Ctrl Pts',(-19.9950718525411,-66.9532260839772,
63.4016368988591));
#180698=CARTESIAN_POINT('Ctrl Pts',(-20.0644762246894,-67.038950459557,
63.5037451943941));
#180699=CARTESIAN_POINT('Ctrl Pts',(-20.1338805884022,-67.1246744025685,
63.6058538308434));
#180700=CARTESIAN_POINT('Ctrl Pts',(-25.3005363491459,-75.4572485563053,
59.89500391474));
#180701=CARTESIAN_POINT('Ctrl Pts',(-25.2707446824789,-74.0955822183551,
59.84745347843));
#180702=CARTESIAN_POINT('Ctrl Pts',(-25.2111613491459,-71.357545302109,
60.18062740255));
#180703=CARTESIAN_POINT('Ctrl Pts',(-25.1217863491459,-67.601945364152,
61.91693136384));
#180704=CARTESIAN_POINT('Ctrl Pts',(-25.0324113491459,-64.56063017797,64.722158934074));
#180705=CARTESIAN_POINT('Ctrl Pts',(-24.9430363491459,-62.52715042104,68.325482238879));
#180706=CARTESIAN_POINT('Ctrl Pts',(-24.8536613491459,-61.69784272518,72.3790257123511));
#180707=CARTESIAN_POINT('Ctrl Pts',(-24.7642863491459,-62.15276622603,76.491447312794));
#180708=CARTESIAN_POINT('Ctrl Pts',(-24.6749113491459,-63.84800247215,80.265720932952));
#180709=CARTESIAN_POINT('Ctrl Pts',(-24.5855363491449,-66.619887661413,
83.33746628068));
#180710=CARTESIAN_POINT('Ctrl Pts',(-24.4961613491449,-70.200815347859,
85.41012737455));
#180711=CARTESIAN_POINT('Ctrl Pts',(-24.4067863491449,-74.2450714527984,
86.28360297416));
#180712=CARTESIAN_POINT('Ctrl Pts',(-24.3174113491449,-78.362210742274,
85.87356499026));
#180713=CARTESIAN_POINT('Ctrl Pts',(-24.2280363491449,-82.154751601322,
84.21959978308));
#180714=CARTESIAN_POINT('Ctrl Pts',(-24.1386613491449,-85.25655017356,81.481386370637));
#180715=CARTESIAN_POINT('Ctrl Pts',(-24.0492863491449,-87.3681490411,77.923280512555));
#180716=CARTESIAN_POINT('Ctrl Pts',(-23.9599113491449,-88.28568778894,73.8887929712529));
#180717=CARTESIAN_POINT('Ctrl Pts',(-23.8705363491449,-87.92058433229,69.767425899435));
#180718=CARTESIAN_POINT('Ctrl Pts',(-23.7811613491449,-86.30808691046,65.957069073716));
#180719=CARTESIAN_POINT('Ctrl Pts',(-23.6917863491449,-83.603871110638,
62.82558636057));
#180720=CARTESIAN_POINT('Ctrl Pts',(-23.6024113491449,-80.069010455704,
60.67530097837));
#180721=CARTESIAN_POINT('Ctrl Pts',(-23.5130363491449,-76.044771542844,
59.71380826027));
#180722=CARTESIAN_POINT('Ctrl Pts',(-23.4236613491449,-71.919667089848,
60.03393374599));
#180723=CARTESIAN_POINT('Ctrl Pts',(-23.3342863491449,-68.091947691899,
61.60477151142));
#180724=CARTESIAN_POINT('Ctrl Pts',(-23.2449113491459,-64.93115345296,64.274667923988));
#180725=CARTESIAN_POINT('Ctrl Pts',(-23.1555363491459,-62.74243741855,67.785862762707));
#180726=CARTESIAN_POINT('Ctrl Pts',(-23.0661613491459,-61.73710513821,71.799374202937));
#180727=CARTESIAN_POINT('Ctrl Pts',(-22.9767863491459,-62.01221456129,75.927725190932));
#180728=CARTESIAN_POINT('Ctrl Pts',(-22.8874113491459,-63.54120575633,79.77235170078));
#180729=CARTESIAN_POINT('Ctrl Pts',(-22.7980363491459,-66.176465090666,
82.962081362607));
#180730=CARTESIAN_POINT('Ctrl Pts',(-22.7086613491459,-69.663576316097,
85.1889676139));
#180731=CARTESIAN_POINT('Ctrl Pts',(-22.6192863491459,-73.665882715971,
86.23801983199));
#180732=CARTESIAN_POINT('Ctrl Pts',(-22.5299113491459,-77.796989006481,
86.00795920683));
#180733=CARTESIAN_POINT('Ctrl Pts',(-22.4405363491459,-81.65806515612,84.52099651684));
#180734=CARTESIAN_POINT('Ctrl Pts',(-22.3511613491459,-84.876350694903,
81.920687830243));
#180735=CARTESIAN_POINT('Ctrl Pts',(-22.2617863491459,-87.14114218589,78.458075149464));
#180736=CARTESIAN_POINT('Ctrl Pts',(-22.1724113491459,-88.233789515,74.467450024384));
#180737=CARTESIAN_POINT('Ctrl Pts',(-22.0830363491459,-88.04880506268,70.334079991696));
#180738=CARTESIAN_POINT('Ctrl Pts',(-21.9936613491459,-86.60404781143,66.457013631716));
#180739=CARTESIAN_POINT('Ctrl Pts',(-21.9042863491459,-84.038999183303,
63.210555159771));
#180740=CARTESIAN_POINT('Ctrl Pts',(-21.8149113491459,-80.601297063461,
60.90812791663));
#180741=CARTESIAN_POINT('Ctrl Pts',(-21.7255363491459,-76.622828057659,
59.7720154906));
#180742=CARTESIAN_POINT('Ctrl Pts',(-21.6361613491459,-72.487686112493,
59.91190175878));
#180743=CARTESIAN_POINT('Ctrl Pts',(-21.5467863491459,-68.595090874297,
61.31428165962));
#180744=CARTESIAN_POINT('Ctrl Pts',(-21.4574113491459,-65.320845765281,
63.843765014137));
#180745=CARTESIAN_POINT('Ctrl Pts',(-21.3680363491459,-62.9810567358,67.256147520865));
#180746=CARTESIAN_POINT('Ctrl Pts',(-21.2786613491459,-61.80161439886,71.22198700936));
#180747=CARTESIAN_POINT('Ctrl Pts',(-21.1892863491459,-61.89638583783,75.358408826466));
#180748=CARTESIAN_POINT('Ctrl Pts',(-21.0999113491459,-63.25622151907,79.266069762973));
#180749=CARTESIAN_POINT('Ctrl Pts',(-21.0105363491459,-65.74983861675,82.567711906636));
#180750=CARTESIAN_POINT('Ctrl Pts',(-20.9211613491459,-69.136495470965,
84.94458431096));
#180751=CARTESIAN_POINT('Ctrl Pts',(-20.8317863491459,-73.089233546913,
86.16721621697));
#180752=CARTESIAN_POINT('Ctrl Pts',(-20.7424113491459,-77.226443043123,
86.11757088408));
#180753=CARTESIAN_POINT('Ctrl Pts',(-20.6530363491459,-81.148704705378,
84.80044122928));
#180754=CARTESIAN_POINT('Ctrl Pts',(-20.5636613491459,-84.477351021258,
82.34298710401));
#180755=CARTESIAN_POINT('Ctrl Pts',(-20.4742863491459,-86.89102397653,78.982458880342));
#180756=CARTESIAN_POINT('Ctrl Pts',(-20.3849113491459,-88.15669997012,75.043292554251));
#180757=CARTESIAN_POINT('Ctrl Pts',(-20.2955363491459,-88.15218665258,70.905787661752));
#180758=CARTESIAN_POINT('Ctrl Pts',(-20.2061613491459,-86.87791974211,66.969391997631));
#180759=CARTESIAN_POINT('Ctrl Pts',(-20.1167863491459,-84.456921029265,
63.614137533019));
#180760=CARTESIAN_POINT('Ctrl Pts',(-20.0274113491459,-81.122921202634,
61.16395142431));
#180761=CARTESIAN_POINT('Ctrl Pts',(-19.9380363491459,-77.19779573134,59.85538121976));
#180762=CARTESIAN_POINT('Ctrl Pts',(-19.8486613491459,-73.060486332881,
59.81476469495));
#180763=CARTESIAN_POINT('Ctrl Pts',(-19.7592863491459,-69.110430400585,
61.04600712199));
#180764=CARTESIAN_POINT('Ctrl Pts',(-19.6699113491459,-65.728947092449,
63.430300094054));
#180765=CARTESIAN_POINT('Ctrl Pts',(-19.6103280158119,-64.07139155217,65.634922657953));
#180766=CARTESIAN_POINT('Ctrl Pts',(-19.5805363491459,-63.431738269,66.837935516246));
#180767=CARTESIAN_POINT('Ctrl Pts',(-25.4573543187099,-75.4467352742876,
60.19606492144));
#180768=CARTESIAN_POINT('Ctrl Pts',(-25.4275626520429,-74.1163770334926,
60.14960778797));
#180769=CARTESIAN_POINT('Ctrl Pts',(-25.3679793187099,-71.441294398629,
60.47512121458));
#180770=CARTESIAN_POINT('Ctrl Pts',(-25.2786043187099,-67.772045047785,
62.1715032276));
#180771=CARTESIAN_POINT('Ctrl Pts',(-25.1892293187099,-64.80065726501,64.912231636138));
#180772=CARTESIAN_POINT('Ctrl Pts',(-25.0998543187099,-62.81393226732,68.432705572515));
#180773=CARTESIAN_POINT('Ctrl Pts',(-25.0104793187089,-62.00369241884,72.393047995661));
#180774=CARTESIAN_POINT('Ctrl Pts',(-24.9211043187089,-62.44815609648,76.41091479114));
#180775=CARTESIAN_POINT('Ctrl Pts',(-24.8317293187089,-64.10441464328,80.098408469768));
#180776=CARTESIAN_POINT('Ctrl Pts',(-24.7423543187089,-66.812567295151,
83.09952674895));
#180777=CARTESIAN_POINT('Ctrl Pts',(-24.6529793187089,-70.311160544158,
85.12453220716));
#180778=CARTESIAN_POINT('Ctrl Pts',(-24.5636043187089,-74.2624291384832,
85.97792442938));
#180779=CARTESIAN_POINT('Ctrl Pts',(-24.4742293187089,-78.284905151586,
85.57731423897));
#180780=CARTESIAN_POINT('Ctrl Pts',(-24.3848543187089,-81.99024605983,83.96137780724));
#180781=CARTESIAN_POINT('Ctrl Pts',(-24.2954793187089,-85.02072656512,81.286122734268));
#180782=CARTESIAN_POINT('Ctrl Pts',(-24.2061043187089,-87.08377452069,77.809826583006));
#180783=CARTESIAN_POINT('Ctrl Pts',(-24.1167293187089,-87.98021676974,73.8681019487348));
#180784=CARTESIAN_POINT('Ctrl Pts',(-24.0273543187089,-87.62350794999,69.841495360525));
#180785=CARTESIAN_POINT('Ctrl Pts',(-23.9379793187089,-86.04808585604,66.118748119013));
#180786=CARTESIAN_POINT('Ctrl Pts',(-23.8486043187089,-83.406046705982,
63.059265985079));
#180787=CARTESIAN_POINT('Ctrl Pts',(-23.7592293187089,-79.952461292809,
60.95842101407));
#180788=CARTESIAN_POINT('Ctrl Pts',(-23.6698543187089,-76.020749645512,
60.01903540591));
#180789=CARTESIAN_POINT('Ctrl Pts',(-23.5804793187089,-71.990491607817,
60.33180041019));
#180790=CARTESIAN_POINT('Ctrl Pts',(-23.4911043187089,-68.250781002811,
61.8665207069));
#180791=CARTESIAN_POINT('Ctrl Pts',(-23.4017293187089,-65.162661287992,
64.475029557805));
#180792=CARTESIAN_POINT('Ctrl Pts',(-23.3123543187089,-63.02426928109,67.905493290763));
#180793=CARTESIAN_POINT('Ctrl Pts',(-23.2229793187089,-62.04205209131,71.826724116717));
#180794=CARTESIAN_POINT('Ctrl Pts',(-23.1336043187099,-62.31083606423,75.860154043494));
#180795=CARTESIAN_POINT('Ctrl Pts',(-23.0442293187099,-63.80467194732,79.616383023829));
#180796=CARTESIAN_POINT('Ctrl Pts',(-22.9548543187099,-66.379340112614,
82.732772864167));
#180797=CARTESIAN_POINT('Ctrl Pts',(-22.8654793187099,-69.786273974476,
84.90845745969));
#180798=CARTESIAN_POINT('Ctrl Pts',(-22.7761043187099,-73.696557391833,
85.93338935707));
#180799=CARTESIAN_POINT('Ctrl Pts',(-22.6867293187099,-77.732679269865,
85.70861839811));
#180800=CARTESIAN_POINT('Ctrl Pts',(-22.5973543187099,-81.504979671842,
84.25584468017));
#180801=CARTESIAN_POINT('Ctrl Pts',(-22.5079793187099,-84.649268818474,
81.715323560263));
#180802=CARTESIAN_POINT('Ctrl Pts',(-22.4186043187099,-86.86198711791,78.332324960555));
#180803=CARTESIAN_POINT('Ctrl Pts',(-22.3292293187099,-87.92951176624,74.43345423642));
#180804=CARTESIAN_POINT('Ctrl Pts',(-22.2398543187099,-87.74878056675,70.395120665275));
#180805=CARTESIAN_POINT('Ctrl Pts',(-22.1504793187099,-86.3372418795,66.607197707679));
#180806=CARTESIAN_POINT('Ctrl Pts',(-22.0611043187099,-83.831170101586,
63.435383393718));
#180807=CARTESIAN_POINT('Ctrl Pts',(-21.9717293187099,-80.472509307037,
61.18589468171));
#180808=CARTESIAN_POINT('Ctrl Pts',(-21.8823543187099,-76.585515202752,
60.07590430719));
#180809=CARTESIAN_POINT('Ctrl Pts',(-21.7929793187099,-72.545450459805,
60.212574242));
#180810=CARTESIAN_POINT('Ctrl Pts',(-21.7036043187099,-68.742355671542,
61.58270993957));
#180811=CARTESIAN_POINT('Ctrl Pts',(-21.6142293187099,-65.543393604434,
64.054034178009));
#180812=CARTESIAN_POINT('Ctrl Pts',(-21.5248543187099,-63.25740214652,67.387957520349));
#180813=CARTESIAN_POINT('Ctrl Pts',(-21.4354793187099,-62.10507812355,71.262612491355));
#180814=CARTESIAN_POINT('Ctrl Pts',(-21.3461043187099,-62.19767053133,75.3039276788));
#180815=CARTESIAN_POINT('Ctrl Pts',(-21.2567293187099,-63.52624020677,79.121741767484));
#180816=CARTESIAN_POINT('Ctrl Pts',(-21.1673543187099,-65.96252284285,82.347470943245));
#180817=CARTESIAN_POINT('Ctrl Pts',(-21.0779793187099,-69.271312029438,
84.66969313695));
#180818=CARTESIAN_POINT('Ctrl Pts',(-20.9886043187099,-73.133166821969,
85.86421369334));
#180819=CARTESIAN_POINT('Ctrl Pts',(-20.8992293187099,-77.175251577815,
85.81570983017));
#180820=CARTESIAN_POINT('Ctrl Pts',(-20.8098543187099,-81.007330685234,
84.52886426336));
#180821=CARTESIAN_POINT('Ctrl Pts',(-20.7204793187099,-84.259443140101,
82.127913122978));
#180822=CARTESIAN_POINT('Ctrl Pts',(-20.6311043187099,-86.61761974852,78.844651804709));
#180823=CARTESIAN_POINT('Ctrl Pts',(-20.5417293187099,-87.85419470181,74.996056713737));
#180824=CARTESIAN_POINT('Ctrl Pts',(-20.4523543187099,-87.84978515668,70.953683353497));
#180825=CARTESIAN_POINT('Ctrl Pts',(-20.3629793187099,-86.60481681305,67.107795220083));
#180826=CARTESIAN_POINT('Ctrl Pts',(-20.2736043187099,-84.239482884453,
63.829686404028));
#180827=CARTESIAN_POINT('Ctrl Pts',(-20.1842293187099,-80.982140009367,
61.43583617042));
#180828=CARTESIAN_POINT('Ctrl Pts',(-20.0948543187099,-77.147262939005,
60.15735325081));
#180829=CARTESIAN_POINT('Ctrl Pts',(-20.0054793187099,-73.105080577911,
60.11767060096));
#180830=CARTESIAN_POINT('Ctrl Pts',(-19.9161043187099,-69.245846259876,
61.32060370107));
#180831=CARTESIAN_POINT('Ctrl Pts',(-19.8267293187099,-65.942111666671,
63.650075845203));
#180832=CARTESIAN_POINT('Ctrl Pts',(-19.7671459853759,-64.32266745252,65.804008650901));
#180833=CARTESIAN_POINT('Ctrl Pts',(-19.7373543187099,-63.6977213899,66.979361250291));
#180834=CARTESIAN_POINT('Ctrl Pts',(-25.6141722882739,-75.4362219922699,
60.49712592814));
#180835=CARTESIAN_POINT('Ctrl Pts',(-25.5843806216069,-74.1371718486303,
60.45176209751));
#180836=CARTESIAN_POINT('Ctrl Pts',(-25.5247972882739,-71.52504349515,60.76961502662));
#180837=CARTESIAN_POINT('Ctrl Pts',(-25.4354222882739,-67.942144731418,
62.42607509136));
#180838=CARTESIAN_POINT('Ctrl Pts',(-25.3460472882739,-65.04068435206,65.102304338201));
#180839=CARTESIAN_POINT('Ctrl Pts',(-25.2566722882729,-63.10071411361,68.539928906151));
#180840=CARTESIAN_POINT('Ctrl Pts',(-25.1672972882729,-62.3095421125,72.4070702789702));
#180841=CARTESIAN_POINT('Ctrl Pts',(-25.0779222882729,-62.74354596694,76.330382269486));
#180842=CARTESIAN_POINT('Ctrl Pts',(-24.9885472882729,-64.36082681442,79.931096006583));
#180843=CARTESIAN_POINT('Ctrl Pts',(-24.8991722882729,-67.005246928886,
82.861587217225));
#180844=CARTESIAN_POINT('Ctrl Pts',(-24.8097972882729,-70.421505740455,
84.83893703977));
#180845=CARTESIAN_POINT('Ctrl Pts',(-24.7204222882729,-74.2797868241642,
85.67224588461));
#180846=CARTESIAN_POINT('Ctrl Pts',(-24.6310472882729,-78.207599560894,
85.28106348769));
#180847=CARTESIAN_POINT('Ctrl Pts',(-24.5416722882729,-81.825740518334,
83.70315583141));
#180848=CARTESIAN_POINT('Ctrl Pts',(-24.4522972882729,-84.784902956671,
81.090859097905));
#180849=CARTESIAN_POINT('Ctrl Pts',(-24.3629222882729,-86.79940000028,77.696372653464));
#180850=CARTESIAN_POINT('Ctrl Pts',(-24.2735472882729,-87.67474575053,73.8474109262254));
#180851=CARTESIAN_POINT('Ctrl Pts',(-24.1841722882729,-87.32643156769,69.915564821625));
#180852=CARTESIAN_POINT('Ctrl Pts',(-24.0947972882729,-85.78808480163,66.280427164319));
#180853=CARTESIAN_POINT('Ctrl Pts',(-24.0054222882729,-83.208222301336,
63.292945609594));
#180854=CARTESIAN_POINT('Ctrl Pts',(-23.9160472882729,-79.835912129926,
61.24154104977));
#180855=CARTESIAN_POINT('Ctrl Pts',(-23.8266722882729,-75.9967277481948,
60.32426255155));
#180856=CARTESIAN_POINT('Ctrl Pts',(-23.7372972882729,-72.061316125801,
60.62966707439));
#180857=CARTESIAN_POINT('Ctrl Pts',(-23.6479222882729,-68.409614313737,
62.12826990236));
#180858=CARTESIAN_POINT('Ctrl Pts',(-23.5585472882729,-65.394169123036,
64.675391191609));
#180859=CARTESIAN_POINT('Ctrl Pts',(-23.4691722882729,-63.30610114364,68.0251238188));
#180860=CARTESIAN_POINT('Ctrl Pts',(-23.3797972882729,-62.34699904441,71.854074030477));
#180861=CARTESIAN_POINT('Ctrl Pts',(-23.2904222882729,-62.60945756717,75.792582896034));
#180862=CARTESIAN_POINT('Ctrl Pts',(-23.2010472882729,-64.06813813831,79.460414346857));
#180863=CARTESIAN_POINT('Ctrl Pts',(-23.1116722882729,-66.582215134543,
82.503464365711));
#180864=CARTESIAN_POINT('Ctrl Pts',(-23.0222972882739,-69.908971632833,
84.62794730547));
#180865=CARTESIAN_POINT('Ctrl Pts',(-22.9329222882739,-73.727232067669,
85.62875888215));
#180866=CARTESIAN_POINT('Ctrl Pts',(-22.8435472882739,-77.668369533221,
85.4092775894));
#180867=CARTESIAN_POINT('Ctrl Pts',(-22.7541722882739,-81.351894187539,
83.99069284351));
#180868=CARTESIAN_POINT('Ctrl Pts',(-22.6647972882739,-84.422186942024,
81.509959290305));
#180869=CARTESIAN_POINT('Ctrl Pts',(-22.5754222882739,-86.58283204993,78.206574771673));
#180870=CARTESIAN_POINT('Ctrl Pts',(-22.4860472882739,-87.62523401748,74.399458448487));
#180871=CARTESIAN_POINT('Ctrl Pts',(-22.3966722882739,-87.44875607083,70.456161338886));
#180872=CARTESIAN_POINT('Ctrl Pts',(-22.3072972882739,-86.07043594758,66.757381783671));
#180873=CARTESIAN_POINT('Ctrl Pts',(-22.2179222882739,-83.623341019893,
63.660211627688));
#180874=CARTESIAN_POINT('Ctrl Pts',(-22.1285472882739,-80.343721550643,
61.4636614468));
#180875=CARTESIAN_POINT('Ctrl Pts',(-22.0391722882739,-76.548202347877,
60.37979312378));
#180876=CARTESIAN_POINT('Ctrl Pts',(-21.9497972882739,-72.603214807152,
60.51324672522));
#180877=CARTESIAN_POINT('Ctrl Pts',(-21.8604222882739,-68.889620468817,
61.85113821951));
#180878=CARTESIAN_POINT('Ctrl Pts',(-21.7710472882739,-65.765941443611,
64.264303341857));
#180879=CARTESIAN_POINT('Ctrl Pts',(-21.6816722882739,-63.53374755725,67.519767519802));
#180880=CARTESIAN_POINT('Ctrl Pts',(-21.5922972882739,-62.40854184824,71.303237973316));
#180881=CARTESIAN_POINT('Ctrl Pts',(-21.5029222882739,-62.49895522482,75.2494465311));
#180882=CARTESIAN_POINT('Ctrl Pts',(-21.4135472882739,-63.79625889445,78.977413771966));
#180883=CARTESIAN_POINT('Ctrl Pts',(-21.3241722882739,-66.175207068926,
82.127229979831));
#180884=CARTESIAN_POINT('Ctrl Pts',(-21.2347972882739,-69.406128587882,
84.39480196293));
#180885=CARTESIAN_POINT('Ctrl Pts',(-21.1454222882739,-73.177100096994,
85.5612111697));
#180886=CARTESIAN_POINT('Ctrl Pts',(-21.0560472882739,-77.124060112478,
85.51384877627));
#180887=CARTESIAN_POINT('Ctrl Pts',(-20.9666722882739,-80.865956665065,
84.25728729746));
#180888=CARTESIAN_POINT('Ctrl Pts',(-20.8772972882739,-84.041535258926,
81.912839141965));
#180889=CARTESIAN_POINT('Ctrl Pts',(-20.7879222882739,-86.34421552051,78.706844729098));
#180890=CARTESIAN_POINT('Ctrl Pts',(-20.6985472882739,-87.5516894335,74.948820873245));
#180891=CARTESIAN_POINT('Ctrl Pts',(-20.6091722882739,-87.54738366077,71.001579045262));
#180892=CARTESIAN_POINT('Ctrl Pts',(-20.5197972882739,-86.331713884,67.246198442551));
#180893=CARTESIAN_POINT('Ctrl Pts',(-20.4304222882739,-84.022044739653,
64.045235275048));
#180894=CARTESIAN_POINT('Ctrl Pts',(-20.3410472882739,-80.841358816111,
61.70772091653));
#180895=CARTESIAN_POINT('Ctrl Pts',(-20.2516722882739,-77.096730146679,
60.45932528185));
#180896=CARTESIAN_POINT('Ctrl Pts',(-20.1622972882739,-73.149674822947,
60.42057650697));
#180897=CARTESIAN_POINT('Ctrl Pts',(-20.0729222882739,-69.381262119169,
61.59520028015));
#180898=CARTESIAN_POINT('Ctrl Pts',(-19.9835472882739,-66.155276240892,
63.869851596353));
#180899=CARTESIAN_POINT('Ctrl Pts',(-19.9239639549399,-64.57394335288,65.973094643852));
#180900=CARTESIAN_POINT('Ctrl Pts',(-19.8941722882739,-63.9637045108,67.120786984341));
#180901=CARTESIAN_POINT('Ctrl Pts',(-25.7709902578379,-75.4257087102522,
60.79818693484));
#180902=CARTESIAN_POINT('Ctrl Pts',(-25.7411985911709,-74.1579666637678,
60.75391640706));
#180903=CARTESIAN_POINT('Ctrl Pts',(-25.6816152578379,-71.60879259167,61.06410883866));
#180904=CARTESIAN_POINT('Ctrl Pts',(-25.5922402578369,-68.112244415052,
62.68064695513));
#180905=CARTESIAN_POINT('Ctrl Pts',(-25.5028652578369,-65.280711439107,
65.292377040265));
#180906=CARTESIAN_POINT('Ctrl Pts',(-25.4134902578369,-63.38749595989,68.647152239787));
#180907=CARTESIAN_POINT('Ctrl Pts',(-25.3241152578369,-62.61539180617,72.4210925622802));
#180908=CARTESIAN_POINT('Ctrl Pts',(-25.2347402578369,-63.0389358374,76.249849747832));
#180909=CARTESIAN_POINT('Ctrl Pts',(-25.1453652578369,-64.61723898556,79.7637835434));
#180910=CARTESIAN_POINT('Ctrl Pts',(-25.0559902578369,-67.197926562624,
82.623647685499));
#180911=CARTESIAN_POINT('Ctrl Pts',(-24.9666152578369,-70.531850936755,
84.55334187238));
#180912=CARTESIAN_POINT('Ctrl Pts',(-24.8772402578369,-74.297144509849,
85.36656733984));
#180913=CARTESIAN_POINT('Ctrl Pts',(-24.7878652578369,-78.130293970206,
84.98481273641));
#180914=CARTESIAN_POINT('Ctrl Pts',(-24.6984902578369,-81.661234976842,
83.44493385557));
#180915=CARTESIAN_POINT('Ctrl Pts',(-24.6091152578369,-84.549079348228,
80.895595461536));
#180916=CARTESIAN_POINT('Ctrl Pts',(-24.5197402578369,-86.51502547987,77.582918723914));
#180917=CARTESIAN_POINT('Ctrl Pts',(-24.4303652578369,-87.36927473133,73.8267199037072));
#180918=CARTESIAN_POINT('Ctrl Pts',(-24.3409902578369,-87.02935518539,69.989634282714));
#180919=CARTESIAN_POINT('Ctrl Pts',(-24.2516152578369,-85.52808374721,66.442106209615));
#180920=CARTESIAN_POINT('Ctrl Pts',(-24.1622402578369,-83.01039789668,63.526625234101));
#180921=CARTESIAN_POINT('Ctrl Pts',(-24.0728652578369,-79.719362967031,
61.52466108548));
#180922=CARTESIAN_POINT('Ctrl Pts',(-23.9834902578369,-75.9727058508626,
60.62948969719));
#180923=CARTESIAN_POINT('Ctrl Pts',(-23.8941152578369,-72.132140643769,
60.92753373859));
#180924=CARTESIAN_POINT('Ctrl Pts',(-23.8047402578369,-68.568447624649,
62.39001909784));
#180925=CARTESIAN_POINT('Ctrl Pts',(-23.7153652578369,-65.625676958068,
64.875752825426));
#180926=CARTESIAN_POINT('Ctrl Pts',(-23.6259902578369,-63.58793300618,68.144754346856));
#180927=CARTESIAN_POINT('Ctrl Pts',(-23.5366152578369,-62.65194599751,71.881423944257));
#180928=CARTESIAN_POINT('Ctrl Pts',(-23.4472402578369,-62.90807907012,75.725011748597));
#180929=CARTESIAN_POINT('Ctrl Pts',(-23.3578652578369,-64.3316043293,79.304445669906));
#180930=CARTESIAN_POINT('Ctrl Pts',(-23.2684902578369,-66.785090156491,
82.274155867272));
#180931=CARTESIAN_POINT('Ctrl Pts',(-23.1791152578369,-70.031669291213,
84.34743715126));
#180932=CARTESIAN_POINT('Ctrl Pts',(-23.0897402578369,-73.757906743531,
85.32412840723));
#180933=CARTESIAN_POINT('Ctrl Pts',(-23.0003652578379,-77.604059796605,
85.10993678068));
#180934=CARTESIAN_POINT('Ctrl Pts',(-22.9109902578379,-81.198808703261,
83.72554100684));
#180935=CARTESIAN_POINT('Ctrl Pts',(-22.8216152578379,-84.195105065595,
81.304595020325));
#180936=CARTESIAN_POINT('Ctrl Pts',(-22.7322402578379,-86.30367698195,78.080824582763));
#180937=CARTESIAN_POINT('Ctrl Pts',(-22.6428652578379,-87.32095626873,74.365462660522));
#180938=CARTESIAN_POINT('Ctrl Pts',(-22.5534902578379,-87.1487315749,70.517202012466));
#180939=CARTESIAN_POINT('Ctrl Pts',(-22.4641152578379,-85.80363001565,66.907565859634));
#180940=CARTESIAN_POINT('Ctrl Pts',(-22.3747402578379,-83.415511938176,
63.885039861635));
#180941=CARTESIAN_POINT('Ctrl Pts',(-22.2853652578379,-80.214933794219,
61.74142821188));
#180942=CARTESIAN_POINT('Ctrl Pts',(-22.1959902578379,-76.510889492969,
60.68368194036));
#180943=CARTESIAN_POINT('Ctrl Pts',(-22.1066152578379,-72.660979154464,
60.81391920844));
#180944=CARTESIAN_POINT('Ctrl Pts',(-22.0172402578379,-69.036885266062,
62.11956649947));
#180945=CARTESIAN_POINT('Ctrl Pts',(-21.9278652578379,-65.988489282763,
64.474572505729));
#180946=CARTESIAN_POINT('Ctrl Pts',(-21.8384902578379,-63.81009296796,67.651577519286));
#180947=CARTESIAN_POINT('Ctrl Pts',(-21.7491152578379,-62.71200557292,71.343863455311));
#180948=CARTESIAN_POINT('Ctrl Pts',(-21.6597402578379,-62.80023991832,75.194965383434));
#180949=CARTESIAN_POINT('Ctrl Pts',(-21.5703652578379,-64.06627758214,78.833085776477));
#180950=CARTESIAN_POINT('Ctrl Pts',(-21.4809902578379,-66.387891295025,
81.90698901644));
#180951=CARTESIAN_POINT('Ctrl Pts',(-21.3916152578379,-69.540945146354,
84.11991078892));
#180952=CARTESIAN_POINT('Ctrl Pts',(-21.3022402578379,-73.22103337205,85.25820864606));
#180953=CARTESIAN_POINT('Ctrl Pts',(-21.2128652578379,-77.07286864717,85.21198772236));
#180954=CARTESIAN_POINT('Ctrl Pts',(-21.1234902578379,-80.72458264492,83.98571033155));
#180955=CARTESIAN_POINT('Ctrl Pts',(-21.0341152578379,-83.823627377769,
81.697765160933));
#180956=CARTESIAN_POINT('Ctrl Pts',(-20.9447402578379,-86.0708112925,78.569037653464));
#180957=CARTESIAN_POINT('Ctrl Pts',(-20.8553652578379,-87.24918416519,74.90158503273));
#180958=CARTESIAN_POINT('Ctrl Pts',(-20.7659902578379,-87.24498216486,71.049474737007));
#180959=CARTESIAN_POINT('Ctrl Pts',(-20.6766152578379,-86.05861095495,67.384601665003));
#180960=CARTESIAN_POINT('Ctrl Pts',(-20.5872402578379,-83.804606594842,
64.260784146057));
#180961=CARTESIAN_POINT('Ctrl Pts',(-20.4978652578379,-80.700577622844,
61.97960566264));
#180962=CARTESIAN_POINT('Ctrl Pts',(-20.4084902578379,-77.046197354344,
60.7612973129));
#180963=CARTESIAN_POINT('Ctrl Pts',(-20.3191152578379,-73.194269067977,
60.72348241298));
#180964=CARTESIAN_POINT('Ctrl Pts',(-20.2297402578379,-69.51667797846,61.86979685924));
#180965=CARTESIAN_POINT('Ctrl Pts',(-20.1403652578379,-66.368440815114,
64.089627347503));
#180966=CARTESIAN_POINT('Ctrl Pts',(-20.0807819245039,-64.82521925324,66.1421806368));
#180967=CARTESIAN_POINT('Ctrl Pts',(-20.0509902578369,-64.2296876317,67.262212718386));
#180968=CARTESIAN_POINT('Ctrl Pts',(-29.0130799422609,-77.577883154178,
84.91151378796));
#180969=CARTESIAN_POINT('Ctrl Pts',(-28.9648716383109,-79.584207200809,
84.47771089461));
#180970=CARTESIAN_POINT('Ctrl Pts',(-28.8684550304109,-83.370581098091,
82.576109782766));
#180971=CARTESIAN_POINT('Ctrl Pts',(-28.7238301185509,-86.96373593251,77.331337332641));
#180972=CARTESIAN_POINT('Ctrl Pts',(-28.5792052067009,-87.57149401059,71.003271823318));
#180973=CARTESIAN_POINT('Ctrl Pts',(-28.4345802948509,-85.04290088059,65.170572201634));
#180974=CARTESIAN_POINT('Ctrl Pts',(-28.2899553829909,-80.008640399699,
61.28849282187));
#180975=CARTESIAN_POINT('Ctrl Pts',(-28.1453304711409,-73.724771677726,
60.32557309628));
#180976=CARTESIAN_POINT('Ctrl Pts',(-28.0007055592909,-67.759060181558,
62.52205714543));
#180977=CARTESIAN_POINT('Ctrl Pts',(-27.8560806474309,-63.59991002351,67.329937790089));
#180978=CARTESIAN_POINT('Ctrl Pts',(-27.7114557355809,-62.28499728294,73.5496847895006));
#180979=CARTESIAN_POINT('Ctrl Pts',(-27.5668308237209,-64.14238315408,79.629517497618));
#180980=CARTESIAN_POINT('Ctrl Pts',(-27.4222059118709,-68.708663616781,
84.05256291155));
#180981=CARTESIAN_POINT('Ctrl Pts',(-27.2775810000209,-74.8445856937055,
85.71530411088));
#180982=CARTESIAN_POINT('Ctrl Pts',(-27.1329560881609,-81.019282482511,
84.20289954075));
#180983=CARTESIAN_POINT('Ctrl Pts',(-26.9883311763109,-85.69221308489,79.892682886532));
#180984=CARTESIAN_POINT('Ctrl Pts',(-26.8437062644609,-87.69751608898,73.860021128897));
#180985=CARTESIAN_POINT('Ctrl Pts',(-26.6990813526009,-86.53488331788,67.610018484104));
#180986=CARTESIAN_POINT('Ctrl Pts',(-26.5544564407489,-82.494382996173,
62.70200410244));
#180987=CARTESIAN_POINT('Ctrl Pts',(-26.4098315288959,-76.58408988664,60.36049104895));
#180988=CARTESIAN_POINT('Ctrl Pts',(-26.2652066170419,-70.278578138388,
61.1696694061));
#180989=CARTESIAN_POINT('Ctrl Pts',(-26.1205817051879,-65.151026010211,
64.927655195095));
#180990=CARTESIAN_POINT('Ctrl Pts',(-25.9759567933349,-62.4807196002,70.696858927558));
#180991=CARTESIAN_POINT('Ctrl Pts',(-25.8313318814809,-62.93388049036,77.037907200944));
#180992=CARTESIAN_POINT('Ctrl Pts',(-25.6867069696279,-66.397448396289,
82.368755669438));
#180993=CARTESIAN_POINT('Ctrl Pts',(-25.5420820577749,-72.007288953952,
85.35939726776));
#180994=CARTESIAN_POINT('Ctrl Pts',(-25.3974571459209,-78.363788487576,
85.26368932913));
#180995=CARTESIAN_POINT('Ctrl Pts',(-25.2528322340679,-83.881048421187,
82.105509685936));
#180996=CARTESIAN_POINT('Ctrl Pts',(-25.1082073222149,-87.18255063842,76.672802844726));
#180997=CARTESIAN_POINT('Ctrl Pts',(-24.9635824103609,-87.44460542796,70.320980571748));
#180998=CARTESIAN_POINT('Ctrl Pts',(-24.8189574985079,-84.601792795156,
64.634805721403));
#180999=CARTESIAN_POINT('Ctrl Pts',(-24.6743325866549,-79.363519912305,
61.03282290959));
#181000=CARTESIAN_POINT('Ctrl Pts',(-24.5297076748019,-73.036149856491,
60.4141243606));
#181001=CARTESIAN_POINT('Ctrl Pts',(-24.4332910668999,-69.145620553249,
62.092366244));
#181002=CARTESIAN_POINT('Ctrl Pts',(-24.3850827629489,-67.523679930053,
63.350471861665));
#181003=CARTESIAN_POINT('Ctrl Pts',(-29.1698979118309,-77.641546433683,
85.2059543519));
#181004=CARTESIAN_POINT('Ctrl Pts',(-29.1216896078809,-79.697418563341,
84.76143828298));
#181005=CARTESIAN_POINT('Ctrl Pts',(-29.0252729999709,-83.57730056992,82.812875320713));
#181006=CARTESIAN_POINT('Ctrl Pts',(-28.8806480881209,-87.25919178487,77.438578220143));
#181007=CARTESIAN_POINT('Ctrl Pts',(-28.7360231762609,-87.88195902748,70.954235106618));
#181008=CARTESIAN_POINT('Ctrl Pts',(-28.5913982644109,-85.29091988206,64.977491413082));
#181009=CARTESIAN_POINT('Ctrl Pts',(-28.4467733525609,-80.132333544284,
60.99954038599));
#181010=CARTESIAN_POINT('Ctrl Pts',(-28.3021484407009,-73.693278699863,
60.01284044075));
#181011=CARTESIAN_POINT('Ctrl Pts',(-28.1575235288509,-67.580238276931,
62.26356875528));
#181012=CARTESIAN_POINT('Ctrl Pts',(-28.0128986170009,-63.31837394482,67.190184591183));
#181013=CARTESIAN_POINT('Ctrl Pts',(-27.8682737051409,-61.97098818188,73.5635341660382));
#181014=CARTESIAN_POINT('Ctrl Pts',(-27.7236487932909,-63.87424396596,79.793514132931));
#181015=CARTESIAN_POINT('Ctrl Pts',(-27.5790238814309,-68.553293073323,
84.32579086559));
#181016=CARTESIAN_POINT('Ctrl Pts',(-27.4343989695809,-74.8407475894004,
86.02959504233));
#181017=CARTESIAN_POINT('Ctrl Pts',(-27.2897740577309,-81.167934395797,
84.47984020103));
#181018=CARTESIAN_POINT('Ctrl Pts',(-27.1451491458709,-85.95626746961,80.063178641754));
#181019=CARTESIAN_POINT('Ctrl Pts',(-27.0005242340209,-88.01109334111,73.8815345568893));
#181020=CARTESIAN_POINT('Ctrl Pts',(-26.8558993221709,-86.81974824651,67.477182144676));
#181021=CARTESIAN_POINT('Ctrl Pts',(-26.7112744103109,-82.679463921444,
62.44795967377));
#181022=CARTESIAN_POINT('Ctrl Pts',(-26.5666494984599,-76.623210494983,
60.04862072552));
#181023=CARTESIAN_POINT('Ctrl Pts',(-26.4220245866059,-70.161978129137,
60.87778251281));
#181024=CARTESIAN_POINT('Ctrl Pts',(-26.2773996747519,-64.907796218,64.728575339723));
#181025=CARTESIAN_POINT('Ctrl Pts',(-26.1327747628989,-62.17154404815,70.640255052583));
#181026=CARTESIAN_POINT('Ctrl Pts',(-25.9881498510449,-62.63589617806,77.137901551893));
#181027=CARTESIAN_POINT('Ctrl Pts',(-25.8435249391919,-66.185000191906,
82.600400400082));
#181028=CARTESIAN_POINT('Ctrl Pts',(-25.6989000273379,-71.933381104597,
85.66489874077));
#181029=CARTESIAN_POINT('Ctrl Pts',(-25.5542751154849,-78.446860447733,
85.56682720345));
#181030=CARTESIAN_POINT('Ctrl Pts',(-25.4096502036319,-84.100374369695,
82.330653306324));
#181031=CARTESIAN_POINT('Ctrl Pts',(-25.2650252917779,-87.48341032833,76.763780595904));
#181032=CARTESIAN_POINT('Ctrl Pts',(-25.1204003799249,-87.75193681046,70.25509402282));
#181033=CARTESIAN_POINT('Ctrl Pts',(-24.9757754680719,-84.838918212374,
64.428493669391));
#181034=CARTESIAN_POINT('Ctrl Pts',(-24.8311505562189,-79.471281192081,
60.73755646174));
#181035=CARTESIAN_POINT('Ctrl Pts',(-24.6865256443659,-72.98765070695,60.10357856287));
#181036=CARTESIAN_POINT('Ctrl Pts',(-24.5901090364639,-69.001041077471,
61.82326622784));
#181037=CARTESIAN_POINT('Ctrl Pts',(-24.5419007325129,-67.33904508595,63.112441961868));
#181038=CARTESIAN_POINT('Ctrl Pts',(-29.3267158813909,-77.705209713196,
85.50039491585));
#181039=CARTESIAN_POINT('Ctrl Pts',(-29.2785075774409,-79.810629925882,
85.04516567134));
#181040=CARTESIAN_POINT('Ctrl Pts',(-29.1820909695409,-83.784020041757,
83.04964085865));
#181041=CARTESIAN_POINT('Ctrl Pts',(-29.0374660576809,-87.55464763724,77.545819107633));
#181042=CARTESIAN_POINT('Ctrl Pts',(-28.8928411458309,-88.19242404437,70.905198389902));
#181043=CARTESIAN_POINT('Ctrl Pts',(-28.7482162339709,-85.53893888352,64.784410624515));
#181044=CARTESIAN_POINT('Ctrl Pts',(-28.6035913221209,-80.256026688849,
60.7105879501));
#181045=CARTESIAN_POINT('Ctrl Pts',(-28.4589664102709,-73.661785721975,
59.70010778522));
#181046=CARTESIAN_POINT('Ctrl Pts',(-28.3143414984109,-67.40141637228,62.00508036515));
#181047=CARTESIAN_POINT('Ctrl Pts',(-28.1697165865609,-63.03683786611,67.050431392305));
#181048=CARTESIAN_POINT('Ctrl Pts',(-28.0250916747109,-61.65697908082,73.5773835426106));
#181049=CARTESIAN_POINT('Ctrl Pts',(-27.8804667628509,-63.60610477786,79.957510768277));
#181050=CARTESIAN_POINT('Ctrl Pts',(-27.7358418510009,-68.3979225299,84.59901881965));
#181051=CARTESIAN_POINT('Ctrl Pts',(-27.5912169391409,-74.836909485138,
86.34388597378));
#181052=CARTESIAN_POINT('Ctrl Pts',(-27.4465920272909,-81.316586309122,
84.75678086128));
#181053=CARTESIAN_POINT('Ctrl Pts',(-27.3019671154409,-86.22032185435,80.233674396936));
#181054=CARTESIAN_POINT('Ctrl Pts',(-27.1573422035809,-88.32467059324,73.903047984833));
#181055=CARTESIAN_POINT('Ctrl Pts',(-27.0127172917309,-87.10461317512,67.344345805202));
#181056=CARTESIAN_POINT('Ctrl Pts',(-26.8680923798809,-82.864544846674,
62.19391524507));
#181057=CARTESIAN_POINT('Ctrl Pts',(-26.7234674680209,-76.662331103274,
59.73675040207));
#181058=CARTESIAN_POINT('Ctrl Pts',(-26.5788425561709,-70.045378119837,
60.58589561953));
#181059=CARTESIAN_POINT('Ctrl Pts',(-26.4342176443159,-64.66456642575,64.52949548439));
#181060=CARTESIAN_POINT('Ctrl Pts',(-26.2895927324629,-61.8623684961,70.583651177657));
#181061=CARTESIAN_POINT('Ctrl Pts',(-26.1449678206089,-62.33791186577,77.237895902889));
#181062=CARTESIAN_POINT('Ctrl Pts',(-26.0003429087559,-65.972551987557,
82.832045130756));
#181063=CARTESIAN_POINT('Ctrl Pts',(-25.8557179969019,-71.859473255285,
85.9704002138));
#181064=CARTESIAN_POINT('Ctrl Pts',(-25.7110930850489,-78.529932407928,
85.86996507777));
#181065=CARTESIAN_POINT('Ctrl Pts',(-25.5664681731959,-84.319700318228,
82.555796926686));
#181066=CARTESIAN_POINT('Ctrl Pts',(-25.4218432613419,-87.78427001824,76.854758347052));
#181067=CARTESIAN_POINT('Ctrl Pts',(-25.2772183494889,-88.05926819295,70.189207473868));
#181068=CARTESIAN_POINT('Ctrl Pts',(-25.1325934376359,-85.07604362958,64.222181617367));
#181069=CARTESIAN_POINT('Ctrl Pts',(-24.9879685257829,-79.579042471845,
60.44229001389));
#181070=CARTESIAN_POINT('Ctrl Pts',(-24.8433436139299,-72.939151557407,
59.79303276515));
#181071=CARTESIAN_POINT('Ctrl Pts',(-24.7469270060279,-68.856461601694,
61.55416621167));
#181072=CARTESIAN_POINT('Ctrl Pts',(-24.6987187020769,-67.154410241852,
62.87441206207));
#181073=CARTESIAN_POINT('Ctrl Pts',(-29.4835338509509,-77.7688729927,85.79483547979));
#181074=CARTESIAN_POINT('Ctrl Pts',(-29.4353255470009,-79.923841288414,
85.32889305971));
#181075=CARTESIAN_POINT('Ctrl Pts',(-29.3389089391009,-83.990739513586,
83.2864063966));
#181076=CARTESIAN_POINT('Ctrl Pts',(-29.1942840272509,-87.85010348959,77.653059995135));
#181077=CARTESIAN_POINT('Ctrl Pts',(-29.0496591153909,-88.50288906125,70.856161673202));
#181078=CARTESIAN_POINT('Ctrl Pts',(-28.9050342035409,-85.78695788499,64.591329835963));
#181079=CARTESIAN_POINT('Ctrl Pts',(-28.7604092916909,-80.379719833434,
60.42163551422));
#181080=CARTESIAN_POINT('Ctrl Pts',(-28.6157843798309,-73.630292744112,
59.38737512969));
#181081=CARTESIAN_POINT('Ctrl Pts',(-28.4711594679809,-67.222594467652,
61.74659197501));
#181082=CARTESIAN_POINT('Ctrl Pts',(-28.3265345561209,-62.75530178742,66.9106781934));
#181083=CARTESIAN_POINT('Ctrl Pts',(-28.1819096442709,-61.34296997975,73.5912329191485));
#181084=CARTESIAN_POINT('Ctrl Pts',(-28.0372847324209,-63.33796558974,80.12150740359));
#181085=CARTESIAN_POINT('Ctrl Pts',(-27.8926598205609,-68.242551986442,
84.87224677369));
#181086=CARTESIAN_POINT('Ctrl Pts',(-27.7480349087109,-74.8330713808332,
86.65817690523));
#181087=CARTESIAN_POINT('Ctrl Pts',(-27.6034099968509,-81.465238222408,
85.03372152155));
#181088=CARTESIAN_POINT('Ctrl Pts',(-27.4587850850009,-86.48437623907,80.404170152158));
#181089=CARTESIAN_POINT('Ctrl Pts',(-27.3141601731509,-88.63824784537,73.924561412825));
#181090=CARTESIAN_POINT('Ctrl Pts',(-27.1695352612909,-87.38947810375,67.211509465773));
#181091=CARTESIAN_POINT('Ctrl Pts',(-27.0249103494409,-83.049625771945,
61.9398708164));
#181092=CARTESIAN_POINT('Ctrl Pts',(-26.8802854375909,-76.701451711617,
59.42488007864));
#181093=CARTESIAN_POINT('Ctrl Pts',(-26.7356605257309,-69.928778110586,
60.29400872623));
#181094=CARTESIAN_POINT('Ctrl Pts',(-26.5910356138809,-64.42133663353,64.330415629018));
#181095=CARTESIAN_POINT('Ctrl Pts',(-26.4464107020269,-61.55319294406,70.527047302681));
#181096=CARTESIAN_POINT('Ctrl Pts',(-26.3017857901729,-62.03992755347,77.337890253839));
#181097=CARTESIAN_POINT('Ctrl Pts',(-26.1571608783199,-65.760103783174,
83.0636898614));
#181098=CARTESIAN_POINT('Ctrl Pts',(-26.0125359664659,-71.78556540593,86.27590168681));
#181099=CARTESIAN_POINT('Ctrl Pts',(-25.8679110546129,-78.613004368084,
86.17310295209));
#181100=CARTESIAN_POINT('Ctrl Pts',(-25.7232861427599,-84.539026266736,
82.780940547073));
#181101=CARTESIAN_POINT('Ctrl Pts',(-25.5786612309059,-88.08512970815,76.94573609823));
#181102=CARTESIAN_POINT('Ctrl Pts',(-25.4340363190529,-88.36659957545,70.12332092494));
#181103=CARTESIAN_POINT('Ctrl Pts',(-25.2894114071999,-85.3131690468,64.015869565355));
#181104=CARTESIAN_POINT('Ctrl Pts',(-25.1447864953469,-79.686803751621,
60.14702356604));
#181105=CARTESIAN_POINT('Ctrl Pts',(-25.0001615834929,-72.890652407866,
59.48248696742));
#181106=CARTESIAN_POINT('Ctrl Pts',(-24.9037449755909,-68.711882125916,
61.28506619551));
#181107=CARTESIAN_POINT('Ctrl Pts',(-24.8555366716399,-66.96977539775,62.63638216227));
#181108=CARTESIAN_POINT('Origin',(-18.5675364832709,-75.,72.98888938658));
#181109=CARTESIAN_POINT('Origin',(-16.5675364832709,-75.,72.98888938658));
#221641=UNCERTAINTY_MEASURE_WITH_UNIT(LENGTH_MEASURE(0.01),#221663,
'DISTANCE_ACCURACY_VALUE',
'Maximum model space distance between geometric entities at asserted c
onnectivities');
#221647=UNCERTAINTY_MEASURE_WITH_UNIT(LENGTH_MEASURE(0.01),#221663,
'DISTANCE_ACCURACY_VALUE',
'Maximum model space distance between geometric entities at asserted c
onnectivities');
#221656=(
GEOMETRIC_REPRESENTATION_CONTEXT(3)
GLOBAL_UNCERTAINTY_ASSIGNED_CONTEXT((#221641))
GLOBAL_UNIT_ASSIGNED_CONTEXT((#221663,#221665,#221666))
REPRESENTATION_CONTEXT('','3D')
);
#221662=(
GEOMETRIC_REPRESENTATION_CONTEXT(3)
GLOBAL_UNCERTAINTY_ASSIGNED_CONTEXT((#221647))
GLOBAL_UNIT_ASSIGNED_CONTEXT((#221663,#221665,#221666))
REPRESENTATION_CONTEXT('','3D')
);
#221663=(
LENGTH_UNIT()
NAMED_UNIT(*)
SI_UNIT(.MILLI.,.METRE.)
);
#221665=(
NAMED_UNIT(*)
PLANE_ANGLE_UNIT()
SI_UNIT($,.RADIAN.)
);
#221666=(
NAMED_UNIT(*)
SI_UNIT($,.STERADIAN.)
SOLID_ANGLE_UNIT()
);
#221675=SHAPE_DEFINITION_REPRESENTATION(#221689,#221716);
#221689=PRODUCT_DEFINITION_SHAPE('',$,#221731);
#221716=SHAPE_REPRESENTATION('',(#80796),#221656);
#221722=PRODUCT_DEFINITION_CONTEXT('part definition',#221766,'design');
#221731=PRODUCT_DEFINITION('2026-10-05-23-02-40-799','Coupling Nut (1)',
#221745,#221722);
#221745=PRODUCT_DEFINITION_FORMATION('',$,#221776);
#221766=APPLICATION_CONTEXT(
'Core Data for Automotive Mechanical Design Process');
#221767=PRODUCT_CONTEXT('part definition',#221766,'mechanical');
#221776=PRODUCT('2026-10-05-23-02-40-799','Coupling Nut (1)',$,(#221767));
#221783=PRESENTATION_STYLE_ASSIGNMENT((#221785));
#221785=SURFACE_STYLE_USAGE(.BOTH.,#221787);
#221787=SURFACE_SIDE_STYLE('',(#221789));
#221789=SURFACE_STYLE_FILL_AREA(#221791);
#221791=FILL_AREA_STYLE('Opaque(202,209,238)',(#221793));
#221793=FILL_AREA_STYLE_COLOUR('Opaque(202,209,238)',#221795);
#221795=COLOUR_RGB('Opaque(202,209,238)', 0.09019608, 0.27058824, 0.51372549);
ENDSEC;
END-ISO-10303-21;
